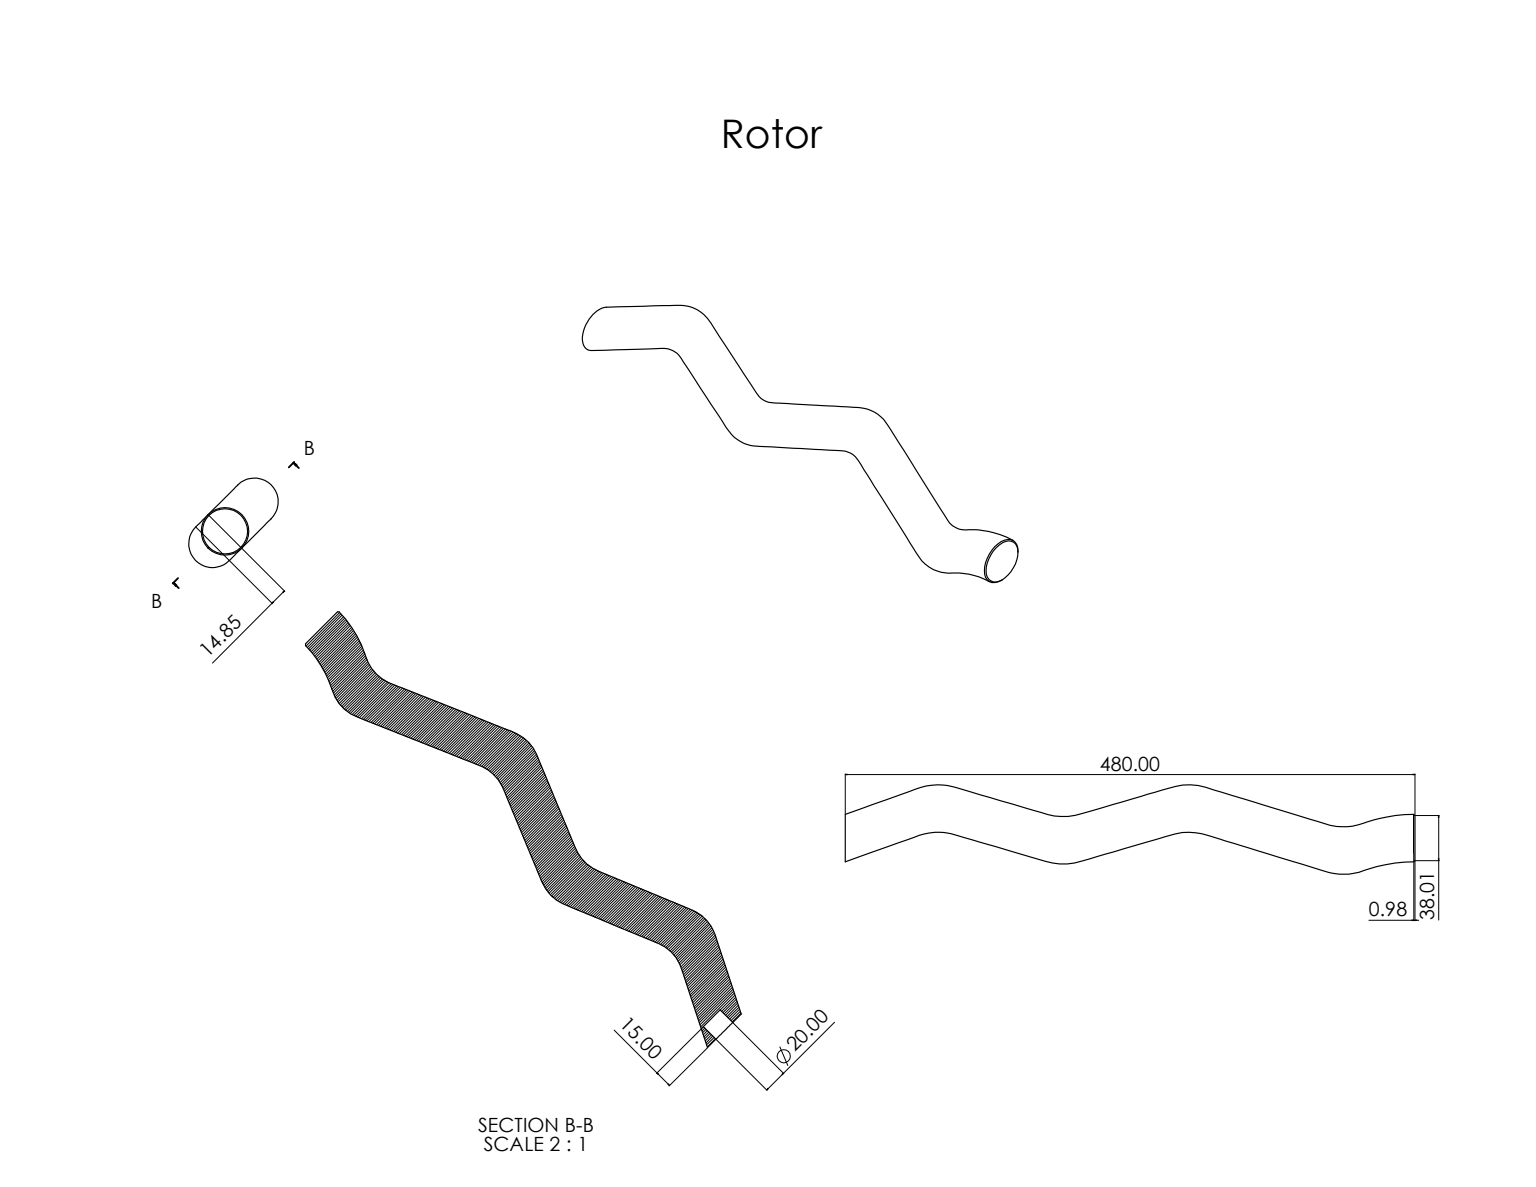
ISO-10303-21;
HEADER;
FILE_DESCRIPTION (('STEP AP214'),
    '1' );
FILE_NAME ('Rotor.step',
    '2026-10-27T19:20:31',
    ( '' ),
    ( '' ),
    'SwSTEP 2.0',
    'SolidWorks 2025',
    '' );
FILE_SCHEMA (( 'AUTOMOTIVE_DESIGN' ));
ENDSEC;

DATA;
#22=DIRECTION ( 'NONE',  ( 0.000000000000000000, 0.000000000000000000, 1.000000000000000000 ) ) ;
#25=CARTESIAN_POINT ( 'NONE',  ( 199.9999999999999432, 19.00168160052138333, -0.2996653188340382967 ) ) ;
#31=CARTESIAN_POINT ( 'NONE',  ( 199.0062801237116332, 7.031410157601610145, -18.72090521856086198 ) ) ;
#36=CARTESIAN_POINT ( 'NONE',  ( 200.0000000000002274, -16.15590588650048787, 10.03807108387658786 ) ) ;
#39=CARTESIAN_POINT ( 'NONE',  ( 199.0246859915949642, -4.071254240408448410, 19.58630271169732140 ) ) ;
#70=CARTESIAN_POINT ( 'NONE',  ( 200.0000000000001421, 16.62132632430557777, -9.210632111445709924 ) ) ;
#71=CARTESIAN_POINT ( 'NONE',  ( 199.9999999999999432, -18.84870794256249482, 2.485603278128234450 ) ) ;
#80=CARTESIAN_POINT ( 'NONE',  ( 199.0199757207951734, 7.646550829590152532, 18.48267855362066214 ) ) ;
#81=CARTESIAN_POINT ( 'NONE',  ( -100.7734535825088358, 12.25131212657497848, -12.25131212657469604 ) ) ;
#83=CARTESIAN_POINT ( 'NONE',  ( 19.06497207195980792, 66.60410523465830579, -10.03556273973354251 ) ) ;
#93=CARTESIAN_POINT ( 'NONE',  ( 199.9999999999998863, -17.04947422730185025, -8.406841951002201441 ) ) ;
#96=CARTESIAN_POINT ( 'NONE',  ( 199.0132273568269170, -10.00203194272371476, -17.32088655864767190 ) ) ;
#122=VERTEX_POINT ( 'NONE', #3583 ) ;
#126=SHAPE_REPRESENTATION ( 'Rotor', ( #21058 ), #20184 ) ;
#127=CARTESIAN_POINT ( 'NONE',  ( 199.9999999999999432, 17.49244587396685091, 7.427265670988617785 ) ) ;
#133=CARTESIAN_POINT ( 'NONE',  ( -259.2033419157646676, 21.55415060305860209, -21.55415060305812602 ) ) ;
#134=CARTESIAN_POINT ( 'NONE',  ( 199.0221265002223845, 3.088699012602908578, 19.76381171561452632 ) ) ;
#159=CARTESIAN_POINT ( 'NONE',  ( 199.9999999999999716, 8.674762155946922348, 16.91470172953081885 ) ) ;
#165=CARTESIAN_POINT ( 'NONE',  ( 199.0071786209885261, 3.739031945787267386, -19.64359944086908527 ) ) ;
#172=CARTESIAN_POINT ( 'NONE',  ( 199.0185982156405089, 10.13449990482401297, 17.24443922940779927 ) ) ;
#197=CARTESIAN_POINT ( 'NONE',  ( 200.0000000000001705, 18.83917254958691601, 2.502331228272203223 ) ) ;
#200=CARTESIAN_POINT ( 'NONE',  ( 199.9999999999999716, -19.00887936793599664, -0.3109487220520843476 ) ) ;
#209=CARTESIAN_POINT ( 'NONE',  ( 199.0242990326260042, -2.747623036511753991, 19.85784534697798875 ) ) ;
#210=CARTESIAN_POINT ( 'NONE',  ( 0.2972598230769959993, 38.42060263243713081, -38.42060263243619289 ) ) ;
#212=CARTESIAN_POINT ( 'NONE',  ( 146.6084372240433709, 3.800685668858042821, 52.76785682606522698 ) ) ;
#224=CARTESIAN_POINT ( 'NONE',  ( 199.0143331921596257, -11.79252763263196613, -16.15335214697885391 ) ) ;
#255=ORIENTED_EDGE ( 'NONE', *, *, #15646, .F. ) ;
#256=CARTESIAN_POINT ( 'NONE',  ( 199.9999999999998295, 18.60987205011830881, -3.837998380785754726 ) ) ;
#263=CARTESIAN_POINT ( 'NONE',  ( -208.1127848780265026, 10.60833733269551615, -10.60833733269529766 ) ) ;
#264=CARTESIAN_POINT ( 'NONE',  ( 199.0256575778758474, -7.963596585350240176, 18.35421432800287533 ) ) ;
#289=CARTESIAN_POINT ( 'NONE',  ( 199.9999999999999716, 17.03617407744741641, 8.421988063785285306 ) ) ;
#298=CARTESIAN_POINT ( 'NONE',  ( 199.0116000645839449, -7.055149577161559549, -18.71482085160166875 ) ) ;
#311=CARTESIAN_POINT ( 'NONE',  ( 199.0082178062215803, 19.99654772287713911, -0.6402344634765599896 ) ) ;
#337=CARTESIAN_POINT ( 'NONE',  ( 199.9999999999997442, 8.817246258963736594, -16.83121203733840332 ) ) ;
#338=CARTESIAN_POINT ( 'NONE',  ( 200.0000000000000284, -8.412522034014145333, -17.05141207210294851 ) ) ;
#349=CARTESIAN_POINT ( 'NONE',  ( 184.8905102610680444, 41.77492675555983936, 14.79361573936436081 ) ) ;
#351=CARTESIAN_POINT ( 'NONE',  ( 0.2972598230769886718, 38.42060263243643448, 18.14793986248763957 ) ) ;
#365=CARTESIAN_POINT ( 'NONE',  ( 199.0262399469797572, -16.26902294624164469, 11.64593733880351500 ) ) ;
#396=CARTESIAN_POINT ( 'NONE',  ( 199.9999999999997726, 10.29466221862743680, -15.97248499526360987 ) ) ;
#403=CARTESIAN_POINT ( 'NONE',  ( 136.1360204305621551, -53.05693388239309627, -3.511608612531332163 ) ) ;
#415=FACE_OUTER_BOUND ( 'NONE', #9966, .T. ) ;
#435=CARTESIAN_POINT ( 'NONE',  ( 199.0205186365099905, -18.88915341724846542, -6.581556047429298673 ) ) ;
#442=STYLED_ITEM('',(#26409),#26080);
#447=CARTESIAN_POINT ( 'NONE',  ( 199.0122446118616892, 18.20979473430505280, 8.267810710173087330 ) ) ;
#461=CARTESIAN_POINT ( 'NONE',  ( 199.0150639398586634, -12.88796719789325707, -15.29887847299889003 ) ) ;
#473=CARTESIAN_POINT ( 'NONE',  ( 199.9999999999999147, 7.974356211459238786, -17.24664066343551028 ) ) ;
#485=CARTESIAN_POINT ( 'NONE',  ( 14.38125909742181463, 10.73282306403652875, -67.30136555895941797 ) ) ;
#487=CARTESIAN_POINT ( 'NONE',  ( 91.82158438592158234, 16.11829626348378142, 40.45024623143977749 ) ) ;
#501=CARTESIAN_POINT ( 'NONE',  ( 200.0000000000000853, -10.31015863810315025, 15.97237410830284254 ) ) ;
#529=CARTESIAN_POINT ( 'NONE',  ( 199.9999999999997442, 17.78964944107278967, -6.681507572083275726 ) ) ;
#534=CARTESIAN_POINT ( 'NONE',  ( -162.0762913951021176, -27.08623940707584055, -29.48230308784799547 ) ) ;
#535=CARTESIAN_POINT ( 'NONE',  ( 199.0191753821509622, 9.128090787448098098, 17.79799345705162139 ) ) ;
#564=CARTESIAN_POINT ( 'NONE',  ( 199.9999999999999147, -2.490047575889294595, 18.88689753006142880 ) ) ;
#570=CARTESIAN_POINT ( 'NONE',  ( 199.0236444319429268, -19.98745889671670284, 0.8241971460415670192 ) ) ;
#581=CARTESIAN_POINT ( 'NONE',  ( 199.0103760074104002, 19.48024492545154018, 4.564568505664855280 ) ) ;
#595=CARTESIAN_POINT ( 'NONE',  ( 199.0058896134214024, 8.852588301136247395, -17.93157114668636964 ) ) ;
#605=CARTESIAN_POINT ( 'NONE',  ( 200.0000000000000000, 15.45062812681867825, -11.05917137904152625 ) ) ;
#616=CARTESIAN_POINT ( 'NONE',  ( 199.0138869583062728, 16.66122972709626637, 11.08110611611319740 ) ) ;
#617=CARTESIAN_POINT ( 'NONE',  ( -280.0000000000000568, -42.42640687119276066, -14.14213562373147148 ) ) ;
#633=CARTESIAN_POINT ( 'NONE',  ( 199.0262887415137527, -15.87643591937917442, 12.17243215972436055 ) ) ;
#660=CARTESIAN_POINT ( 'NONE',  ( 199.9999999999999432, 6.681520191215184035, -17.78964488229654251 ) ) ;
#664=CARTESIAN_POINT ( 'NONE',  ( 199.0161420530203600, 13.89456085230456850, 14.38651294782529888 ) ) ;
#695=CARTESIAN_POINT ( 'NONE',  ( 199.9999999999999147, 3.087032903897462432, 18.75855398088509318 ) ) ;
#701=CARTESIAN_POINT ( 'NONE',  ( 199.0171635947087907, -15.67013318013508716, -12.42972081464992407 ) ) ;
#705=AXIS2_PLACEMENT_3D ( 'NONE', #5212, #19434, #1220 ) ;
#715=CARTESIAN_POINT ( 'NONE',  ( 199.0068072339493597, 19.36029496603142874, -5.002335373038918398 ) ) ;
#731=CARTESIAN_POINT ( 'NONE',  ( 199.0058341074146142, 9.150281110520873895, -17.78147227136547670 ) ) ;
#733=ORIENTED_EDGE ( 'NONE', *, *, #5255, .F. ) ;
#743=CARTESIAN_POINT ( 'NONE',  ( 199.9999999999999432, 6.681520191215184035, -17.78964488229654251 ) ) ;
#744=CARTESIAN_POINT ( 'NONE',  ( 199.9999999999999147, -5.229706238425958276, -18.27161031230872368 ) ) ;
#752=CARTESIAN_POINT ( 'NONE',  ( 199.0072939989582324, 19.72179417679889823, -3.362695692811099590 ) ) ;
#753=CARTESIAN_POINT ( 'NONE',  ( -56.48582580120559271, -6.472252184284276844, 6.472252184284108978 ) ) ;
#767=CARTESIAN_POINT ( 'NONE',  ( 199.0263606093525652, -14.93202714917829965, 13.31409215216611663 ) ) ;
#796=CARTESIAN_POINT ( 'NONE',  ( 200.0000000000003126, 10.03286793820859835, -16.13825081434616493 ) ) ;
#799=CARTESIAN_POINT ( 'NONE',  ( 146.6084372240433709, -52.76785682606510619, -3.800685668859292043 ) ) ;
#800=CARTESIAN_POINT ( 'NONE',  ( 199.0185982156405089, 10.13449990482401297, 17.24443922940779927 ) ) ;
#815=CARTESIAN_POINT ( 'NONE',  ( -280.0000000000000000, -14.14213562373118549, 14.14213562373078936 ) ) ;
#833=CARTESIAN_POINT ( 'NONE',  ( 199.0220583073800640, -19.74674823417053915, -3.257374120286249397 ) ) ;
#844=CARTESIAN_POINT ( 'NONE',  ( 199.0053210531128229, 14.60061869579413063, -13.67646033072836786 ) ) ;
#860=CARTESIAN_POINT ( 'NONE',  ( 199.0089017020823121, -1.168865339877916965, -19.99575268797839911 ) ) ;
#872=CARTESIAN_POINT ( 'NONE',  ( 199.9999999999996021, 9.500464834803043601, -16.45734938164063621 ) ) ;
#873=CARTESIAN_POINT ( 'NONE',  ( 199.9999999999999432, 2.163685940895884841, -18.88015187541845918 ) ) ;
#883=CARTESIAN_POINT ( 'NONE',  ( 199.0119004238765967, 18.48644426806060181, 7.626980851762527713 ) ) ;
#885=CARTESIAN_POINT ( 'NONE',  ( -91.56559293963834989, -16.03295912088728414, 16.03295912088688269 ) ) ;
#898=CARTESIAN_POINT ( 'NONE',  ( 200.0000000000000000, -12.54535540268124372, 14.29661512548269187 ) ) ;
#925=CARTESIAN_POINT ( 'NONE',  ( 199.9999999999999716, -3.557237102606629620, -18.66704445460036865 ) ) ;
#929=CARTESIAN_POINT ( 'NONE',  ( 199.0091071337781159, 19.93120984291649478, 1.649067560610785854 ) ) ;
#943=CARTESIAN_POINT ( 'NONE',  ( 199.0250816517838359, -5.508431349499541163, 19.23181920140171997 ) ) ;
#946=CARTESIAN_POINT ( 'NONE',  ( 151.7948205124836534, 4.785054706297857230, 51.78348778862544322 ) ) ;
#963=CARTESIAN_POINT ( 'NONE',  ( 199.0254590212676078, -18.72437106667806717, 7.049340093992902290 ) ) ;
#990=CARTESIAN_POINT ( 'NONE',  ( 199.0112255263369718, -6.317613805557628304, -18.97682060292212114 ) ) ;
#1000=CARTESIAN_POINT ( 'NONE',  ( 199.9999999999999147, -10.82539530975288855, -15.62049148088690131 ) ) ;
#1010=CARTESIAN_POINT ( 'NONE',  ( -213.1075012329537230, 9.698598906450543566, -9.698598906450348167 ) ) ;
#1027=CARTESIAN_POINT ( 'NONE',  ( 199.9999999999999716, 2.158921371974932057, 18.88613560767030464 ) ) ;
#1051=CARTESIAN_POINT ( 'NONE',  ( 200.0000000000000568, 2.475862818518347552, -18.83975305017670365 ) ) ;
#1055=CARTESIAN_POINT ( 'NONE',  ( 199.0190933210857906, 9.274233341078666371, 17.72222919763310856 ) ) ;
#1069=CARTESIAN_POINT ( 'NONE',  ( 0.2972598230769938343, 10.13633138497486286, -10.13633138497461594 ) ) ;
#1084=CARTESIAN_POINT ( 'NONE',  ( 200.0000000000000568, 3.396018298074437780, 18.70303282425911462 ) ) ;
#1122=CARTESIAN_POINT ( 'NONE',  ( -265.0000000000000000, -4.867971026610730343E-14, -6.532754371361504014E-30 ) ) ;
#1132=CARTESIAN_POINT ( 'NONE',  ( 199.9999999999994031, -18.37269623729978107, -4.912321869774860517 ) ) ;
#1157=CARTESIAN_POINT ( 'NONE',  ( 200.0000000000003695, 4.006257452897062699, 18.58368358710308144 ) ) ;
#1182=CARTESIAN_POINT ( 'NONE',  ( 199.9999999999999147, -13.00175152101318510, -13.87559618198639022 ) ) ;
#1185=CARTESIAN_POINT ( 'NONE',  ( 199.0075387591496110, 2.605640672139595715, -19.82598477556707195 ) ) ;
#1206=( LENGTH_UNIT ( ) NAMED_UNIT ( * ) SI_UNIT ( .MILLI., .METRE. ) );
#1215=CARTESIAN_POINT ( 'NONE',  ( 200.0000000000000853, -10.31015863810315025, 15.97237410830284254 ) ) ;
#1220=DIRECTION ( 'NONE',  ( 0.000000000000000000, -1.000000000000000000, 0.000000000000000000 ) ) ;
#1243=CARTESIAN_POINT ( 'NONE',  ( 199.0233014162839140, -20.00325696956714339, -0.1274617848538161236 ) ) ;
#1251=CARTESIAN_POINT ( 'NONE',  ( 136.1360204305621266, 3.511608612530757068, -3.511608612530642937 ) ) ;
#1253=CARTESIAN_POINT ( 'NONE',  ( 199.9999999999998010, -18.94725682776174835, -1.557189005449375330 ) ) ;
#1277=CARTESIAN_POINT ( 'NONE',  ( 199.9999999999998295, 8.812783067309094776, 16.84096882534935702 ) ) ;
#1304=CARTESIAN_POINT ( 'NONE',  ( 199.9999999999996305, -13.87326568555608830, -12.99368172854615366 ) ) ;
#1307=CARTESIAN_POINT ( 'NONE',  ( 199.0053384867209445, 15.04244419640346031, -13.18878631234924192 ) ) ;
#1328=CARTESIAN_POINT ( 'NONE',  ( -86.96347745069644475, -15.38646221621807442, 15.38646221621768184 ) ) ;
#1333=ORIENTED_EDGE ( 'NONE', *, *, #17104, .F. ) ;
#1339=CARTESIAN_POINT ( 'NONE',  ( 200.0000000000003411, -11.08347333911627963, 15.44584840147742355 ) ) ;
#1349=B_SPLINE_CURVE_WITH_KNOTS ( 'NONE', 3,
 ( #13548, #17297, #15539, #5314, #1457, #9433, #11058, #13425, #21548, #7058, #19543, #17540, #1328, #7425, #25678, #23667, #21301, #5447, #9184, #21801, #9691, #7684, #17797, #23922, #3574, #13679, #15798, #25943, #11677, #19802 ),
 .UNSPECIFIED., .F., .F.,
 ( 4, 2, 2, 2, 2, 2, 2, 2, 2, 2, 2, 2, 2, 2, 4 ),
 ( 0.000000000000000000, 0.1357259735107005372, 0.1651108541090157700, 0.1944957347073310028, 0.3598804999793158710, 0.3867117631979620773, 0.4135430264166082281, 0.5789277916885930964, 0.6062785021374117456, 0.6336292125862302838, 0.8508620842112317728, 0.8814014469398914198, 0.9119408096685510667, 0.9559704048342755334, 0.9981086137545830406 ),
 .UNSPECIFIED. ) ;
#1384=CARTESIAN_POINT ( 'NONE',  ( 199.9999999999999716, -15.72304121538119936, -10.67928908684366540 ) ) ;
#1410=CARTESIAN_POINT ( 'NONE',  ( 200.0000000000000568, -6.707298731100607370, 17.79007541258576452 ) ) ;
#1434=CARTESIAN_POINT ( 'NONE',  ( 200.0000000000000000, -10.04040541317802315, -16.13598245992451297 ) ) ;
#1438=CARTESIAN_POINT ( 'NONE',  ( 199.0055466334479206, 16.72508833076945223, -10.95857635003404873 ) ) ;
#1457=CARTESIAN_POINT ( 'NONE',  ( -208.1127848780265026, 10.60833733269551615, -10.60833733269529766 ) ) ;
#1467=CARTESIAN_POINT ( 'NONE',  ( 199.9999999999998863, -2.178116022715518074, 18.88665387132288487 ) ) ;
#1468=CARTESIAN_POINT ( 'NONE',  ( -280.0000000000000000, 14.14213562373108424, -14.14213562373078759 ) ) ;
#1500=CARTESIAN_POINT ( 'NONE',  ( 199.0198738297864338, -18.40122271749203620, -7.840790799891646401 ) ) ;
#1502=ORIENTED_EDGE ( 'NONE', *, *, #5255, .T. ) ;
#1508=CARTESIAN_POINT ( 'NONE',  ( -208.1127848780265026, 38.89260858015777700, -38.89260858015687461 ) ) ;
#1511=CARTESIAN_POINT ( 'NONE',  ( 199.9999999999998579, -17.31468161508541570, -7.846489601088847188 ) ) ;
#1526=CARTESIAN_POINT ( 'NONE',  ( 184.8905102610680444, -14.79361573936399665, 14.79361573936367158 ) ) ;
#1541=CARTESIAN_POINT ( 'NONE',  ( 199.9999999999998579, 3.088973468740698447, 18.75625871509165776 ) ) ;
#1554=CARTESIAN_POINT ( 'NONE',  ( 57.59792236341147031, 26.56190807104652052, 30.00663442387728708 ) ) ;
#1566=CARTESIAN_POINT ( 'NONE',  ( 200.0000000000000568, -15.63904601878861733, 10.81246610429574595 ) ) ;
#1569=CARTESIAN_POINT ( 'NONE',  ( 199.0059805750804571, 8.391908656364034158, -18.14947886101857932 ) ) ;
#1600=CARTESIAN_POINT ( 'NONE',  ( 199.9999999999996874, -6.995992324030534171, 17.67857064404661926 ) ) ;
#1606=CARTESIAN_POINT ( 'NONE',  ( 0.2972598230769959993, 38.42060263243713081, -38.42060263243619289 ) ) ;
#1642=CARTESIAN_POINT ( 'NONE',  ( 91.82158438592158234, 16.11829626346161604, -16.11829626346121103 ) ) ;
#1660=AXIS2_PLACEMENT_3D ( 'NONE', #24424, #14168, #4078 ) ;
#1671=FACE_OUTER_BOUND ( 'NONE', #18068, .T. ) ;
#1672=CARTESIAN_POINT ( 'NONE',  ( 199.9999999999998863, 18.50936851023984886, -4.296315843485498220 ) ) ;
#1675=CARTESIAN_POINT ( 'NONE',  ( 199.9999999999999432, -18.10102589806735907, -5.808760618774897466 ) ) ;
#1687=CARTESIAN_POINT ( 'NONE',  ( 184.8905102610680444, -14.79361573936399665, 14.79361573936367158 ) ) ;
#1690=CARTESIAN_POINT ( 'NONE',  ( 57.59792236341147031, -1.722363176415055985, 1.722363176415024677 ) ) ;
#1703=CARTESIAN_POINT ( 'NONE',  ( 199.0069448139248891, 19.47830345430216070, -4.521371627647083891 ) ) ;
#1729=CARTESIAN_POINT ( 'NONE',  ( 200.0000000000000284, 10.29196162618721644, 15.98165385515595815 ) ) ;
#1735=CARTESIAN_POINT ( 'NONE',  ( -56.48582580120559982, -6.472252184283581400, -50.09629031063973059 ) ) ;
#1736=CYLINDRICAL_SURFACE ( 'NONE', #23013, 10.00000000000000000 ) ;
#1762=CARTESIAN_POINT ( 'NONE',  ( 200.0000000000000000, 18.75319608166667251, -3.074485549213874069 ) ) ;
#1770=CARTESIAN_POINT ( 'NONE',  ( 199.0064300168743898, 6.416848550863170964, -18.94043562797172697 ) ) ;
#1781=CARTESIAN_POINT ( 'NONE',  ( 199.0160554649137907, 14.01242985958090692, 14.27167877623515757 ) ) ;
#1806=CARTESIAN_POINT ( 'NONE',  ( 199.0053211798077086, 14.13837298227953987, -14.13837298578013701 ) ) ;
#1807=CARTESIAN_POINT ( 'NONE',  ( 199.9999999999999432, 16.89472078740815775, 8.702431973737679627 ) ) ;
#1808=CARTESIAN_POINT ( 'NONE',  ( 199.9999999999999147, -18.88644897276319412, 2.180134100127611330 ) ) ;
#1818=CARTESIAN_POINT ( 'NONE',  ( 199.0148629966199962, 15.54375530361796010, 12.59047442983698417 ) ) ;
#1820=CARTESIAN_POINT ( 'NONE',  ( -100.7734535825088500, -16.03295912088659492, -40.53558337403696044 ) ) ;
#1823=CARTESIAN_POINT ( 'NONE',  ( -192.9588430854689989, 10.23066800230756712, -10.23066800230735396 ) ) ;
#1834=CARTESIAN_POINT ( 'NONE',  ( 199.9999999999999147, -18.99336422956244874, -0.7807574862979690389 ) ) ;
#1837=CARTESIAN_POINT ( 'NONE',  ( 199.0183492910935286, -16.99256592298258184, -10.55490704374186883 ) ) ;
#1867=CARTESIAN_POINT ( 'NONE',  ( 199.9999999999998863, 8.252615397115851792, 17.12261885615216173 ) ) ;
#1873=CARTESIAN_POINT ( 'NONE',  ( -30.26275506840323715, 29.48230279907829754, -29.48230279907758344 ) ) ;
#1874=CARTESIAN_POINT ( 'NONE',  ( 199.0245441510845410, -3.586860678693493565, 19.68275873856094549 ) ) ;
#1898=CARTESIAN_POINT ( 'NONE',  ( 199.9999999999999432, 17.99863635774381621, -6.096428138147773623 ) ) ;
#1905=CARTESIAN_POINT ( 'NONE',  ( 199.0078712948245823, 1.622169390422157242, -19.93073376281416031 ) ) ;
#1912=CARTESIAN_POINT ( 'NONE',  ( 199.0218477376944577, 3.734929907270702287, 19.65178994764128717 ) ) ;
#1939=CARTESIAN_POINT ( 'NONE',  ( 200.0000000000005116, 16.46820326627658204, -9.481692438271846157 ) ) ;
#1940=CARTESIAN_POINT ( 'NONE',  ( 199.9999999999999432, -18.70500695855449891, 3.403006402435800215 ) ) ;
#1943=CARTESIAN_POINT ( 'NONE',  ( -100.7734535825088500, -16.03295912088659492, -40.53558337403696044 ) ) ;
#1950=CARTESIAN_POINT ( 'NONE',  ( 199.0255783348552825, -7.592917736791534367, 18.50773992579789251 ) ) ;
#1951=CARTESIAN_POINT ( 'NONE',  ( 200.0000000000000000, 42.42640687119267540, 14.14213562373153543 ) ) ;
#1966=CARTESIAN_POINT ( 'NONE',  ( 200.0000000000001137, -18.36608873747554327, 4.914565663504686377 ) ) ;
#1970=CARTESIAN_POINT ( 'NONE',  ( 199.0201284062958962, -18.60237515726647572, -7.352601386804158423 ) ) ;
#1987=SHAPE_DEFINITION_REPRESENTATION ( #9744, #126 ) ;
#1996=CARTESIAN_POINT ( 'NONE',  ( 199.9999999999995737, 11.06459441337805494, 15.46579378046570952 ) ) ;
#2004=CARTESIAN_POINT ( 'NONE',  ( 184.8905102610680444, -14.79361573936330565, -41.77492675556016621 ) ) ;
#2005=CARTESIAN_POINT ( 'NONE',  ( 199.0247325273615502, -4.232801689760709252, 19.55205092890061280 ) ) ;
#2034=CARTESIAN_POINT ( 'NONE',  ( 199.9999999999999432, 12.28098720308154945, 14.50824971548827946 ) ) ;
#2040=CARTESIAN_POINT ( 'NONE',  ( 199.0075387591496110, 2.605640672139595715, -19.82598477556707195 ) ) ;
#2045=CARTESIAN_POINT ( 'NONE',  ( 200.0000000000001990, -15.46007656673369368, 11.06691610098113543 ) ) ;
#2048=CARTESIAN_POINT ( 'NONE',  ( 199.0248683625651154, -4.715036670046848677, 19.44145415004932076 ) ) ;
#2072=DIRECTION ( 'NONE',  ( -1.000000000000000000, -1.836970198721030181E-16, -2.465190328815661892E-32 ) ) ;
#2073=CARTESIAN_POINT ( 'NONE',  ( 199.9999999999999716, 17.67160698027466736, 6.995183481556395577 ) ) ;
#2074=CARTESIAN_POINT ( 'NONE',  ( 199.9999999999998863, -18.51554692031677973, -4.309913066855557418 ) ) ;
#2083=CARTESIAN_POINT ( 'NONE',  ( 199.0253317321493398, -6.507757088401906032, 18.91903323328891062 ) ) ;
#2085=CARTESIAN_POINT ( 'NONE',  ( -238.4067589809705794, 0.6820004458491113475, -57.25054294077229144 ) ) ;
#2087=CARTESIAN_POINT ( 'NONE',  ( -162.0762913951021176, 57.76657433523994456, -1.198031840315424867 ) ) ;
#2096=CARTESIAN_POINT ( 'NONE',  ( 199.9999999999998579, -15.18157530797039101, 11.44282300742696457 ) ) ;
#2100=CARTESIAN_POINT ( 'NONE',  ( 199.0125641721520822, -8.847877585088737007, -17.93749959268865979 ) ) ;
#2119=ORIENTED_EDGE ( 'NONE', *, *, #8406, .T. ) ;
#2128=CARTESIAN_POINT ( 'NONE',  ( 199.9999999999999432, 17.03543292729471403, 8.423468753378063667 ) ) ;
#2134=CARTESIAN_POINT ( 'NONE',  ( -135.8532207217289738, 21.81201906317798134, -21.81201906317747685 ) ) ;
#2135=CARTESIAN_POINT ( 'NONE',  ( 199.0258842571097375, -9.142960865851959440, 17.79628948870135829 ) ) ;
#2162=CARTESIAN_POINT ( 'NONE',  ( 200.0000000000000000, 9.495512316542487952, 16.46764514154290637 ) ) ;
#2169=CARTESIAN_POINT ( 'NONE',  ( 199.0057329523134513, 9.713090712928652337, -17.48024697358846069 ) ) ;
#2176=CARTESIAN_POINT ( 'NONE',  ( 199.9999999999998863, -17.44218472118251384, 7.566354988273278792 ) ) ;
#2179=CARTESIAN_POINT ( 'NONE',  ( 199.0212010157159455, 5.167062836304152640, 19.32642926518865423 ) ) ;
#2206=CARTESIAN_POINT ( 'NONE',  ( 199.9999999999997442, 18.75350838795884201, -3.072479883316599381 ) ) ;
#2207=CARTESIAN_POINT ( 'NONE',  ( 199.9999999999999147, -11.57906590988528528, -15.07304842808868273 ) ) ;
#2210=CARTESIAN_POINT ( 'NONE',  ( -280.0000000000000000, -5.143516556418885689E-14, 0.000000000000000000 ) ) ;
#2216=CARTESIAN_POINT ( 'NONE',  ( 199.0260505877926960, -10.07036125175988772, 17.33556466753674385 ) ) ;
#2217=CARTESIAN_POINT ( 'NONE',  ( 19.06497207195980792, 66.60410523465830579, -10.03556273973354251 ) ) ;
#2219=CARTESIAN_POINT ( 'NONE',  ( -198.0356074513804572, 39.15871834505887250, 17.40982414986519089 ) ) ;
#2231=CARTESIAN_POINT ( 'NONE',  ( 199.0178460907175690, -16.45326163792621443, -11.37340206338170923 ) ) ;
#2258=CARTESIAN_POINT ( 'NONE',  ( 200.0000000000001137, 17.30391983412833667, 7.856783789979721710 ) ) ;
#2264=CARTESIAN_POINT ( 'NONE',  ( 4.995406935893294431, -17.50105314357144337, -39.06748935135212264 ) ) ;
#2265=DIRECTION ( 'NONE',  ( -1.000000000000000000, -1.836970198721030181E-16, -2.465190328815661892E-32 ) ) ;
#2280=EDGE_LOOP ( 'NONE', ( #12322, #25337 ) ) ;
#2288=CARTESIAN_POINT ( 'NONE',  ( 199.9999999999999147, 18.96428544249645043, -1.225771028434774923 ) ) ;
#2293=CARTESIAN_POINT ( 'NONE',  ( 199.0060750228415429, 7.941611777091910795, -18.35102805502410561 ) ) ;
#2297=CARTESIAN_POINT ( 'NONE',  ( -280.0000000000000000, -5.143516556418885689E-14, 0.000000000000000000 ) ) ;
#2303=CARTESIAN_POINT ( 'NONE',  ( 199.0201394418415077, 7.332745681712491859, 18.61237044096938575 ) ) ;
#2331=CARTESIAN_POINT ( 'NONE',  ( 200.0000000000000000, 2.939587388390868306, -18.77290383772223592 ) ) ;
#2332=CARTESIAN_POINT ( 'NONE',  ( 199.9999999999999716, -2.174716591481574035, -18.87967999152925103 ) ) ;
#2343=CARTESIAN_POINT ( 'NONE',  ( 199.0193791362118532, 8.756460839110824068, 17.98522136602180055 ) ) ;
#2344=CARTESIAN_POINT ( 'NONE',  ( 4.995406935893286438, 67.35176059880245703, -10.78321810387767066 ) ) ;
#2346=CARTESIAN_POINT ( 'NONE',  ( -100.7734535825088500, 12.25131212657428748, 44.31723036834913643 ) ) ;
#2360=CARTESIAN_POINT ( 'NONE',  ( 199.0130599948309680, -9.716555752287060699, -17.48250520384952367 ) ) ;
#2388=CARTESIAN_POINT ( 'NONE',  ( 199.9999999999996021, 4.009690090792337180, -18.57554820616829261 ) ) ;
#2394=CARTESIAN_POINT ( 'NONE',  ( 184.8905102610680444, -43.07788698682556827, -13.49065550809859104 ) ) ;
#2395=CARTESIAN_POINT ( 'NONE',  ( 199.0262120803540995, -11.39568569719682145, 16.44280778893389439 ) ) ;
#2408=CARTESIAN_POINT ( 'NONE',  ( 199.0261461916015264, -10.84957391917088110, 16.80813345823991867 ) ) ;
#2422=CARTESIAN_POINT ( 'NONE',  ( 199.9999999999999716, -6.125576256895536531, 18.00661530747469996 ) ) ;
#2428=CARTESIAN_POINT ( 'NONE',  ( 199.0198127172867828, -18.35326955327933618, -7.958687714023728432 ) ) ;
#2436=CARTESIAN_POINT ( 'NONE',  ( -265.0000000000000000, -4.867971026610730343E-14, -6.532754371361504014E-30 ) ) ;
#2437=CARTESIAN_POINT ( 'NONE',  ( 199.0066757862822726, 19.23093628729661475, -5.478378800400602877 ) ) ;
#2450=APPLICATION_CONTEXT ( 'automotive_design' ) ;
#2452=CARTESIAN_POINT ( 'NONE',  ( 199.0118788846117468, -7.586312082139164303, -18.50318004405354699 ) ) ;
#2464=CARTESIAN_POINT ( 'NONE',  ( 200.0000000000001137, 15.89309473284322749, -10.41337480477382371 ) ) ;
#2474=CARTESIAN_POINT ( 'NONE',  ( 199.0112297511867325, 18.97400286213774834, 6.326091761587574247 ) ) ;
#2475=CARTESIAN_POINT ( 'NONE',  ( 163.1118516004056573, -47.56205970284945295, -9.006482792074823607 ) ) ;
#2477=CARTESIAN_POINT ( 'NONE',  ( 0.2972598230769907257, 66.70487387989869887, -10.13633138497392494 ) ) ;
#2493=CARTESIAN_POINT ( 'NONE',  ( 199.9999999999997158, -10.44119114510941770, 15.88703355754643098 ) ) ;
#2523=CARTESIAN_POINT ( 'NONE',  ( 199.9999999999998863, 12.52392839731578889, -14.30162278802013098 ) ) ;
#2526=CARTESIAN_POINT ( 'NONE',  ( 130.8568914410475372, -24.07718906447255947, 24.07718906447199458 ) ) ;
#2527=CARTESIAN_POINT ( 'NONE',  ( 199.0117592729713465, 18.59672480091233737, 7.361113620700817428 ) ) ;
#2554=CARTESIAN_POINT ( 'NONE',  ( 199.9999999999999716, -10.82917866272351581, 15.62749623992054637 ) ) ;
#2561=CARTESIAN_POINT ( 'NONE',  ( 199.0234688043258018, -20.00162938710794691, 0.3307560783973806373 ) ) ;
#2575=CARTESIAN_POINT ( 'NONE',  ( 199.0055623607443636, 10.83365079593514757, -16.80863377785637169 ) ) ;
#2590=CARTESIAN_POINT ( 'NONE',  ( 199.0118983629657237, -7.623092896147099395, -18.48804935406682404 ) ) ;
#2602=CARTESIAN_POINT ( 'NONE',  ( 199.9999999999997726, 7.546454185142647653, -17.43816512261951956 ) ) ;
#2603=CARTESIAN_POINT ( 'NONE',  ( 199.9999999999999147, 4.913383178421502073, -18.36491317384603761 ) ) ;
#2613=CARTESIAN_POINT ( 'NONE',  ( 199.0063941363436584, 18.94647080546362261, -6.505566240119136090 ) ) ;
#2614=CARTESIAN_POINT ( 'NONE',  ( 130.8568914410475088, -52.36146031193413108, -4.207082182990267150 ) ) ;
#2633=CARTESIAN_POINT ( 'NONE',  ( 199.0262772983307400, -15.97594543884460450, 12.04151787815577102 ) ) ;
#2663=CARTESIAN_POINT ( 'NONE',  ( 199.9999999999999147, 7.974356211459238786, -17.24664066343551028 ) ) ;
#2668=CARTESIAN_POINT ( 'NONE',  ( 199.0194208361885444, 8.684746017668368623, 18.01861981654000999 ) ) ;
#2695=( NAMED_UNIT ( * ) SI_UNIT ( $, .STERADIAN. ) SOLID_ANGLE_UNIT ( ) );
#2698=CARTESIAN_POINT ( 'NONE',  ( 199.9999999999999432, 5.207736135262080346, 18.28309964035191726 ) ) ;
#2704=CARTESIAN_POINT ( 'NONE',  ( 199.0181825105790665, -16.81808889125263207, -10.83063377519274795 ) ) ;
#2715=CARTESIAN_POINT ( 'NONE',  ( 199.0093797572272081, 19.86600527971208763, 2.306481033292959726 ) ) ;
#2729=CARTESIAN_POINT ( 'NONE',  ( 199.0053214113103763, 13.24708851623085870, -15.02902163144573500 ) ) ;
#2740=CARTESIAN_POINT ( 'NONE',  ( 199.9999999999997726, -2.174764995058875439, -18.87968408895515182 ) ) ;
#2741=CARTESIAN_POINT ( 'NONE',  ( 200.0000000000000000, -0.6316560126811792131, -18.99370827960111541 ) ) ;
#2750=CARTESIAN_POINT ( 'NONE',  ( 199.0114847477458397, 18.79655487626452981, 6.828771775710518632 ) ) ;
#2752=CARTESIAN_POINT ( 'NONE',  ( -238.4067589809705794, -27.60227080167029001, -28.96627169325357798 ) ) ;
#2766=CARTESIAN_POINT ( 'NONE',  ( 199.0230409161751197, -19.98726064469808961, -0.8218112272605428981 ) ) ;
#2793=CARTESIAN_POINT ( 'NONE',  ( 199.9999999999999716, 18.70067531203203970, -3.379044910449504169 ) ) ;
#2796=CARTESIAN_POINT ( 'NONE',  ( 0.2972598230769938343, 10.13633138497486286, -10.13633138497461594 ) ) ;
#2797=CARTESIAN_POINT ( 'NONE',  ( 199.0206025836015442, 6.413712542583970944, 18.94893284924772203 ) ) ;
#2834=CARTESIAN_POINT ( 'NONE',  ( 199.0145894657785846, -12.18649378798404470, -15.86093292504746621 ) ) ;
#2848=CARTESIAN_POINT ( 'NONE',  ( 199.0060751070798233, 18.35498561216385482, -7.937441424495496278 ) ) ;
#2874=CARTESIAN_POINT ( 'NONE',  ( 199.9999999999997726, 10.29466221862743680, -15.97248499526360987 ) ) ;
#2875=CARTESIAN_POINT ( 'NONE',  ( 199.9999999999999147, -6.120187099840395106, -17.99310556315726117 ) ) ;
#2883=CARTESIAN_POINT ( 'NONE',  ( 199.0060844782017000, 18.36908416490651064, -7.898827608825804703 ) ) ;
#2884=CARTESIAN_POINT ( 'NONE',  ( 170.2234770963711128, -17.36149277826940462, -39.20704971665412586 ) ) ;
#2898=CARTESIAN_POINT ( 'NONE',  ( 199.0254590212676078, -18.72437106667806717, 7.049340093992902290 ) ) ;
#2922=CARTESIAN_POINT ( 'NONE',  ( 199.9999999999999147, -6.121038220875967717, -17.99280653461927315 ) ) ;
#2926=CARTESIAN_POINT ( 'NONE',  ( 199.0173417939125784, 12.16728005963107329, 15.88742495833056800 ) ) ;
#2940=CARTESIAN_POINT ( 'NONE',  ( -100.7734535825088358, -16.03295912088728770, 16.03295912088687913 ) ) ;
#2952=CARTESIAN_POINT ( 'NONE',  ( 199.9999999999999716, -11.08296553609489798, 15.44857252758585631 ) ) ;
#2956=CARTESIAN_POINT ( 'NONE',  ( 199.0186803405091780, -17.32754287553631301, -9.995805879000721816 ) ) ;
#2986=CARTESIAN_POINT ( 'NONE',  ( 199.0053211804427633, 14.13331159297750617, -14.14343255912447361 ) ) ;
#2998=CARTESIAN_POINT ( 'NONE',  ( 200.0000000000000284, -14.89093438834758842, -11.81132417993805639 ) ) ;
#3007=CARTESIAN_POINT ( 'NONE',  ( 199.0094106630088220, 19.89429631425563372, 2.408647560944259691 ) ) ;
#3009=CARTESIAN_POINT ( 'NONE',  ( 170.2234770963711128, -45.64576402573167258, -10.92277846919254891 ) ) ;
#3023=CARTESIAN_POINT ( 'NONE',  ( 199.0053211798077086, 14.13837298227953987, -14.13837298578013701 ) ) ;
#3024=CARTESIAN_POINT ( 'NONE',  ( 200.0000000000001421, -10.70065846580424207, 15.71346033962178446 ) ) ;
#3047=CARTESIAN_POINT ( 'NONE',  ( 199.9999999999999147, 0.2978356717867484682, -19.00168788844713319 ) ) ;
#3050=CARTESIAN_POINT ( 'NONE',  ( 199.0082178062215803, 19.99654772287713911, -0.6402344634765599896 ) ) ;
#3067=CARTESIAN_POINT ( 'NONE',  ( 199.0258313909553749, -8.851116586292111066, 17.94317422212728630 ) ) ;
#3069=CARTESIAN_POINT ( 'NONE',  ( -213.1075012329537230, 37.98287015391211696, 18.58567234101190735 ) ) ;
#3086=CARTESIAN_POINT ( 'NONE',  ( 199.0263606093525652, -14.93202714917829965, 13.31409215216611663 ) ) ;
#3105=ORIENTED_EDGE ( 'NONE', *, *, #16287, .F. ) ;
#3111=CARTESIAN_POINT ( 'NONE',  ( 199.0230723762332161, -19.99042835476056368, -0.7383407320838223376 ) ) ;
#3122=CARTESIAN_POINT ( 'NONE',  ( 199.9999999999999716, -17.78976893299991247, -6.695511796223322598 ) ) ;
#3132=B_SPLINE_CURVE_WITH_KNOTS ( 'NONE', 3,
 ( #11253, #9647, #7634, #20030, #7906, #20159, #9911, #18285, #15883, #10316, #18017, #16025, #4211, #10181, #18422, #10048, #16297, #7768, #24295, #5789, #22434, #1940, #18154, #71, #1808, #26166, #12301, #200, #11907, #8307, #22298, #20428, #6185, #22167, #14165, #2074, #24009, #21886, #1675, #26301, #4074, #24150, #26031, #6313, #5927, #3942, #14034, #13896, #8044, #12039, #22030, #16432, #19890, #16160, #3663, #6063, #3803, #12176, #20297, #9780, #2207, #8180, #24421, #24558, #14300, #11771, #17882, #8848, #338, #16828, #12844, #4868, #2875, #10983, #744, #12565, #14962, #16691, #21095, #4734, #20960, #2332, #10575, #8442, #2741, #19093, #12972, #16958, #873, #14433, #8713, #23097, #22562, #6577, #2603, #24824, #18690, #12433, #18559, #25096, #8982, #6843, #17089, #10845, #25221, #4341, #16561, #24690, #20561, #10445, #20699, #12701, #6446, #14696, #14562 ),
 .UNSPECIFIED., .F., .F.,
 ( 4, 2, 1, 2, 2, 2, 2, 2, 1, 2, 2, 2, 2, 2, 2, 1, 2, 2, 2, 2, 2, 1, 2, 2, 2, 2, 2, 2, 2, 2, 2, 2, 2, 2, 1, 2, 2, 2, 2, 2, 2, 2, 2, 2, 2, 2, 2, 1, 2, 2, 2, 2, 2, 1, 2, 2, 2, 2, 2, 2, 4 ),
 ( 0.000000000000000000, 0.01562500000000010061, 0.02343750000000014572, 0.02734375000000015613, 0.03125000000000015959, 0.04687500000000018041, 0.05468750000000021511, 0.06250000000000024980, 0.07031250000000029143, 0.07421875000000027756, 0.07812500000000027756, 0.09375000000000033307, 0.1015625000000003608, 0.1093750000000003886, 0.1250000000000004441, 0.1328125000000004718, 0.1367187500000004718, 0.1406250000000004718, 0.1562500000000004996, 0.1640625000000005274, 0.1718750000000005551, 0.1796875000000005829, 0.1835937500000006106, 0.1875000000000006106, 0.2031250000000007494, 0.2109375000000008049, 0.2187500000000008604, 0.2265625000000009159, 0.2343750000000009437, 0.2421875000000009992, 0.2500000000000010547, 0.2656250000000012768, 0.2734375000000013878, 0.2812500000000014988, 0.2890625000000015543, 0.2929687500000015543, 0.2968750000000015543, 0.3125000000000014988, 0.3203125000000014433, 0.3281250000000013878, 0.3359375000000013323, 0.3437500000000012768, 0.3515625000000012212, 0.3593750000000011657, 0.3671875000000011102, 0.3750000000000009992, 0.3906250000000009437, 0.3984375000000008882, 0.4023437500000008882, 0.4062500000000008327, 0.4218750000000006661, 0.4296875000000005551, 0.4375000000000004441, 0.4453125000000003886, 0.4492187500000003331, 0.4531250000000003331, 0.4609375000000002220, 0.4687500000000001665, 0.4765625000000001110, 0.4843750000000000555, 0.5000000000000000000 ),
 .UNSPECIFIED. ) ;
#3148=CARTESIAN_POINT ( 'NONE',  ( 199.9999999999999716, 1.225499021177249404, 18.97167928969624384 ) ) ;
#3174=CARTESIAN_POINT ( 'NONE',  ( 199.9999999999999147, -4.475453068641236598, -18.46865746885900705 ) ) ;
#3177=CARTESIAN_POINT ( 'NONE',  ( 199.0073806320087613, 3.093635517344801578, -19.75563546371214230 ) ) ;
#3202=CARTESIAN_POINT ( 'NONE',  ( 199.0263771353516233, -14.14574067859894413, 14.14574067859863682 ) ) ;
#3235=CARTESIAN_POINT ( 'NONE',  ( 199.0255658961882830, -18.53135165341859292, 7.535237739358464637 ) ) ;
#3246=CARTESIAN_POINT ( 'NONE',  ( 200.0000000000001137, -7.564955314186367907, -17.43543124971759539 ) ) ;
#3274=CARTESIAN_POINT ( 'NONE',  ( 199.9999999999999716, 8.673909288817675645, 16.91296503504769078 ) ) ;
#3301=CARTESIAN_POINT ( 'NONE',  ( 199.9999999999998579, -2.482523633563583410, -18.84177167654976515 ) ) ;
#3304=CARTESIAN_POINT ( 'NONE',  ( 199.0057363775755448, 17.49143510765091492, -9.692886659233986180 ) ) ;
#3331=CARTESIAN_POINT ( 'NONE',  ( 199.0262110011730954, -16.45735938206000171, 11.37817034370231006 ) ) ;
#3355=CARTESIAN_POINT ( 'NONE',  ( 200.0000000000000000, -13.44239485489230290, 13.44239485489200803 ) ) ;
#3358=CARTESIAN_POINT ( 'NONE',  ( 199.0193679503813939, -17.97530889761664596, -8.776769756081623797 ) ) ;
#3369=CARTESIAN_POINT ( 'NONE',  ( 199.9999999999998863, -11.82502131081330887, -14.88093782183822888 ) ) ;
#3393=DIRECTION ( 'NONE',  ( -1.000000000000000000, -1.836970198721030181E-16, -2.465190328815661892E-32 ) ) ;
#3399=CARTESIAN_POINT ( 'NONE',  ( 200.0000000000000000, 5.800536564436440834, 18.10358378745109320 ) ) ;
#3413=CARTESIAN_POINT ( 'NONE',  ( -259.2033419157646676, -6.730120644403663199, 6.730120644403451813 ) ) ;
#3422=CARTESIAN_POINT ( 'NONE',  ( 199.9999999999999147, -15.08385563027219156, -11.56407354529143205 ) ) ;
#3426=CARTESIAN_POINT ( 'NONE',  ( 199.0066333181452478, 19.18530965003537858, -5.635992787424102701 ) ) ;
#3459=CARTESIAN_POINT ( 'NONE',  ( 200.0000000000000853, -13.44239485489230290, 13.44239485489200803 ) ) ;
#3504=CARTESIAN_POINT ( 'NONE',  ( 200.0000000000001705, -16.91021041590709473, -8.683373960011902426 ) ) ;
#3528=CARTESIAN_POINT ( 'NONE',  ( 200.0000000000000284, 12.51656570147539327, 14.30544205704861760 ) ) ;
#3541=CARTESIAN_POINT ( 'NONE',  ( -91.56559293963834989, -16.03295912088728414, 16.03295912088688269 ) ) ;
#3553=CARTESIAN_POINT ( 'NONE',  ( 200.0000000000002274, -18.85575486854367355, -2.482946933799725642 ) ) ;
#3556=CARTESIAN_POINT ( 'NONE',  ( 199.0060750228415429, 7.941611777091910795, -18.35102805502410561 ) ) ;
#3574=CARTESIAN_POINT ( 'NONE',  ( 151.7948205124836250, -23.49921654116371883, 23.49921654116317526 ) ) ;
#3583=CARTESIAN_POINT ( 'NONE',  ( -280.0000000000000000, -10.00000000000005151, -6.902532920683853297E-30 ) ) ;
#3585=CARTESIAN_POINT ( 'NONE',  ( 200.0000000000005684, -1.253076495463282924, 18.97792690268338234 ) ) ;
#3590=CARTESIAN_POINT ( 'NONE',  ( -30.26275506840324070, 1.198031551616724366, -57.76657404653984429 ) ) ;
#3618=CARTESIAN_POINT ( 'NONE',  ( 199.0253302299943812, -18.92118621875344786, 6.501515187515664707 ) ) ;
#3632=CARTESIAN_POINT ( 'NONE',  ( 200.0000000000000853, -13.44239485489230290, 13.44239485489200803 ) ) ;
#3648=CARTESIAN_POINT ( 'NONE',  ( 146.6084372240433993, -24.48358557860353457, 24.48358557860296258 ) ) ;
#3662=CARTESIAN_POINT ( 'NONE',  ( 199.9999999999998579, -4.480715147297966716, 18.47471730767352938 ) ) ;
#3663=CARTESIAN_POINT ( 'NONE',  ( 199.9999999999999716, -14.29283438936585604, -12.53096660533077689 ) ) ;
#3675=CARTESIAN_POINT ( 'NONE',  ( 14.38125909742180220, 39.01709431150892016, 17.55144818341517166 ) ) ;
#3678=CARTESIAN_POINT ( 'NONE',  ( -280.0000000000000000, -14.14213562373118549, 14.14213562373078936 ) ) ;
#3693=CARTESIAN_POINT ( 'NONE',  ( 199.0058097323984327, 9.278912463403225175, -17.71230630396810213 ) ) ;
#3724=CARTESIAN_POINT ( 'NONE',  ( 199.9999999999998863, 18.69362872516077800, 3.425107952296777114 ) ) ;
#3730=CARTESIAN_POINT ( 'NONE',  ( 57.59792236341147031, 26.56190807104720975, -26.56190807104655249 ) ) ;
#3755=CARTESIAN_POINT ( 'NONE',  ( 199.9999999999999716, 18.51141176942600097, 4.336711825884415283 ) ) ;
#3761=CARTESIAN_POINT ( 'NONE',  ( 199.0074854128475579, 2.768696461275208520, -19.80384161416936806 ) ) ;
#3766=CARTESIAN_POINT ( 'NONE',  ( -135.8532207217289738, 21.81201906317798134, -21.81201906317747685 ) ) ;
#3768=CARTESIAN_POINT ( 'NONE',  ( 200.0000000000001705, -18.10265802883496278, 5.810802590798905598 ) ) ;
#3771=CARTESIAN_POINT ( 'NONE',  ( 199.0206025836015442, 6.413712542583970944, 18.94893284924772203 ) ) ;
#3802=CARTESIAN_POINT ( 'NONE',  ( 199.9999999999999716, 18.70067531203203970, -3.379044910449504169 ) ) ;
#3803=CARTESIAN_POINT ( 'NONE',  ( 200.0000000000000000, -13.65901895451712811, -13.21854774209566585 ) ) ;
#3814=CARTESIAN_POINT ( 'NONE',  ( 199.0150730930814689, 15.28768747664870453, 12.90128171110900013 ) ) ;
#3816=CARTESIAN_POINT ( 'NONE',  ( -105.3755690713226585, 41.18208027870575449, 15.38646221621837107 ) ) ;
#3829=CARTESIAN_POINT ( 'NONE',  ( 199.9999999999999716, -18.76480772196043034, -3.095184993347289026 ) ) ;
#3832=CARTESIAN_POINT ( 'NONE',  ( 199.0093721751683518, -2.288394243462712030, -19.86801947894618792 ) ) ;
#3860=CARTESIAN_POINT ( 'NONE',  ( 200.0000000000000568, 5.208214048020466613, 18.28294570233482119 ) ) ;
#3868=CARTESIAN_POINT ( 'NONE',  ( -238.4067589809705794, 0.6820004458491113475, -57.25054294077229144 ) ) ;
#3869=CARTESIAN_POINT ( 'NONE',  ( 199.0251223662492635, -5.665586242881555101, 19.18612710904600149 ) ) ;
#3888=ORIENTED_EDGE ( 'NONE', *, *, #19870, .T. ) ;
#3899=CARTESIAN_POINT ( 'NONE',  ( 199.9999999999999716, 18.84369875136934880, -2.460375794728051790 ) ) ;
#3906=CARTESIAN_POINT ( 'NONE',  ( 199.0059208051008852, 8.690306674284110855, -18.00847358856242408 ) ) ;
#3915=CARTESIAN_POINT ( 'NONE',  ( 199.0173417939125784, 12.16728005963107329, 15.88742495833056800 ) ) ;
#3941=CARTESIAN_POINT ( 'NONE',  ( 199.9999999999999432, 18.93973332185608172, 1.567235916626209535 ) ) ;
#3942=CARTESIAN_POINT ( 'NONE',  ( 199.9999999999999716, -16.61824216245382502, -9.229554904678261451 ) ) ;
#3951=CARTESIAN_POINT ( 'NONE',  ( 199.0221514193071926, 3.032938341077176414, 19.78261031040590012 ) ) ;
#3952=CARTESIAN_POINT ( 'NONE',  ( 4.995406935893290878, 39.06748935135239265, -39.06748935135144762 ) ) ;
#3966=CARTESIAN_POINT ( 'NONE',  ( 199.9999999999998579, -18.00099009291985297, -6.105420735363839668 ) ) ;
#3971=CARTESIAN_POINT ( 'NONE',  ( 199.0198127172867828, -18.35326955327933618, -7.958687714023728432 ) ) ;
#3997=CARTESIAN_POINT ( 'NONE',  ( 199.9999999999998579, 13.86282612285610938, 13.00154682524819805 ) ) ;
#4003=CARTESIAN_POINT ( 'NONE',  ( -86.96347745069644475, -15.38646221621738164, -41.18208027870615240 ) ) ;
#4004=CARTESIAN_POINT ( 'NONE',  ( 199.0220573263155188, 3.250837537642027542, 19.73775173755759127 ) ) ;
#4031=CARTESIAN_POINT ( 'NONE',  ( 199.9999999999999147, 15.61914218176268143, 10.83067004454828641 ) ) ;
#4038=CARTESIAN_POINT ( 'NONE',  ( 199.0065087001378572, 6.107362818253672998, -19.04251412529381327 ) ) ;
#4046=CARTESIAN_POINT ( 'NONE',  ( 199.0161420530203600, 13.89456085230456850, 14.38651294782529888 ) ) ;
#4073=CARTESIAN_POINT ( 'NONE',  ( 200.0000000000000853, 16.14603016630555743, -10.01676266068942667 ) ) ;
#4074=CARTESIAN_POINT ( 'NONE',  ( 199.9999999999998863, -17.79060443684709369, -6.693342262146931176 ) ) ;
#4078=DIRECTION ( 'NONE',  ( 0.000000000000000000, -0.7071067811865561215, 0.7071067811865389130 ) ) ;
#4084=CARTESIAN_POINT ( 'NONE',  ( 199.0206793870229376, 6.297627498482031072, 19.03991857512456320 ) ) ;
#4085=CARTESIAN_POINT ( 'NONE',  ( 14.38125909742181108, 39.01709431150961649, -39.01709431150867147 ) ) ;
#4088=CARTESIAN_POINT ( 'NONE',  ( 19.06497207195979726, 38.31983398719604139, 18.24870850772803976 ) ) ;
#4098=CARTESIAN_POINT ( 'NONE',  ( 200.0000000000000853, -13.44239485489230290, 13.44239485489200803 ) ) ;
#4101=CARTESIAN_POINT ( 'NONE',  ( 199.0111317961331281, -6.131174403448985011, -19.03732645848564431 ) ) ;
#4135=CARTESIAN_POINT ( 'NONE',  ( 199.9999999999998863, 12.28125103214278901, 14.50804496155330447 ) ) ;
#4143=CARTESIAN_POINT ( 'NONE',  ( -280.0000000000000000, 14.14213562373108246, -14.14213562373078581 ) ) ;
#4144=CARTESIAN_POINT ( 'NONE',  ( 199.0262541782678340, -11.79586192385960430, 16.15815307234555576 ) ) ;
#4169=CARTESIAN_POINT ( 'NONE',  ( 199.9999999999999716, 16.82248425547956217, 8.841323171526189739 ) ) ;
#4175=CARTESIAN_POINT ( 'NONE',  ( 199.0087111817176435, -0.6649071253763039202, -19.99597453042600392 ) ) ;
#4180=CARTESIAN_POINT ( 'NONE',  ( 200.0000000000000284, -14.89458464808834748, 11.81399803044240038 ) ) ;
#4183=CARTESIAN_POINT ( 'NONE',  ( 199.0152755141893692, 15.03153897770602221, 13.19647528785794677 ) ) ;
#4209=CARTESIAN_POINT ( 'NONE',  ( 200.0000000000001421, 16.60215271479902910, 9.252637072649047667 ) ) ;
#4211=CARTESIAN_POINT ( 'NONE',  ( 199.9999999999999147, -17.31672820518381783, 7.849270303112303004 ) ) ;
#4221=CARTESIAN_POINT ( 'NONE',  ( 199.0168430542531155, 12.91005451537445126, 15.29445721284177573 ) ) ;
#4224=CARTESIAN_POINT ( 'NONE',  ( -192.9588430854690273, 10.23066800229588758, -66.79921049721882298 ) ) ;
#4226=CARTESIAN_POINT ( 'NONE',  ( 136.1360204305621551, 31.79587985999232558, 24.77266263493161702 ) ) ;
#4239=CARTESIAN_POINT ( 'NONE',  ( 199.0181825105790665, -16.81808889125263207, -10.83063377519274795 ) ) ;
#4266=CARTESIAN_POINT ( 'NONE',  ( 199.9999999999998863, 17.10417011681778732, 8.282922153951966848 ) ) ;
#4272=CARTESIAN_POINT ( 'NONE',  ( 0.2972598230769990524, -18.14793986248671231, -38.42060263243687501 ) ) ;
#4273=CARTESIAN_POINT ( 'NONE',  ( 199.0263771353516233, -14.14574067859894413, 14.14574067859863682 ) ) ;
#4289=CARTESIAN_POINT ( 'NONE',  ( -208.1127848780265026, 10.60833733269551615, -10.60833733269529766 ) ) ;
#4301=CARTESIAN_POINT ( 'NONE',  ( 200.0000000000000000, 6.097653648161206696, 18.01359495397503352 ) ) ;
#4308=CARTESIAN_POINT ( 'NONE',  ( 199.0137359473271488, -10.84478214295758036, -16.80398351328055639 ) ) ;
#4317=CARTESIAN_POINT ( 'NONE',  ( 199.0145894300637792, 15.86095929198710586, 12.18642508278280623 ) ) ;
#4340=CARTESIAN_POINT ( 'NONE',  ( 199.9999999999998863, -5.231270638550959085, -18.27112563740264761 ) ) ;
#4341=CARTESIAN_POINT ( 'NONE',  ( 199.9999999999999716, 9.498725063112413380, -16.45837312633763005 ) ) ;
#4350=CARTESIAN_POINT ( 'NONE',  ( 199.0255859347418834, -7.628281087858428400, 18.49319637005222816 ) ) ;
#4351=CARTESIAN_POINT ( 'NONE',  ( -280.0000000000000568, -14.14213562373049449, -42.42640687119305198 ) ) ;
#4353=CARTESIAN_POINT ( 'NONE',  ( 184.8905102610680444, 41.77492675555983936, 14.79361573936436081 ) ) ;
#4368=CARTESIAN_POINT ( 'NONE',  ( 199.0152737994447136, -13.19951906643276374, -15.03942049639883294 ) ) ;
#4384=B_SPLINE_CURVE_WITH_KNOTS ( 'NONE', 3,
 ( #21596, #15590, #25478, #17850, #1508, #15345, #5496, #9483, #3766, #17719, #19463, #17587, #19594, #7605, #15719, #17464, #13863, #21856, #19856, #11737, #1642, #26000, #1251, #23978, #9355, #25607, #7350, #15463, #23590, #5369 ),
 .UNSPECIFIED., .F., .F.,
 ( 4, 2, 2, 2, 2, 2, 2, 2, 2, 2, 2, 2, 2, 2, 4 ),
 ( 0.000000000000000000, 0.1357259735107005372, 0.1651108541090157700, 0.1944957347073310028, 0.3598804999793158710, 0.3867117631979620773, 0.4135430264166082281, 0.5789277916885930964, 0.6062785021374117456, 0.6336292125862302838, 0.8508620842112317728, 0.8814014469398914198, 0.9119408096685510667, 0.9559704048342755334, 0.9980677081714144361 ),
 .UNSPECIFIED. ) ;
#4394=CARTESIAN_POINT ( 'NONE',  ( 199.9999999999998579, 18.23094931701148269, -5.355502299499542040 ) ) ;
#4399=CARTESIAN_POINT ( 'NONE',  ( 184.8905102610680444, -14.79361573936399665, 14.79361573936367158 ) ) ;
#4400=CARTESIAN_POINT ( 'NONE',  ( 199.0242446922718784, -2.616032970993653173, 19.83497009005848710 ) ) ;
#4413=CARTESIAN_POINT ( 'NONE',  ( -135.8532207217289738, -6.472252184284280396, 6.472252184284099208 ) ) ;
#4424=CARTESIAN_POINT ( 'NONE',  ( 200.0000000000000284, 4.307699855108636733, 18.51410484079663377 ) ) ;
#4430=CARTESIAN_POINT ( 'NONE',  ( 199.0232879746372134, -20.00360196692749071, -0.1645009869758431997 ) ) ;
#4440=CARTESIAN_POINT ( 'NONE',  ( 199.0089741461167989, 19.95552976068599804, 1.321036586804004820 ) ) ;
#4448=DIRECTION ( 'NONE',  ( -1.000000000000000000, -1.836970198721030181E-16, -2.465190328815661892E-32 ) ) ;
#4456=CARTESIAN_POINT ( 'NONE',  ( 199.0061375790170644, 7.656915158548016187, -18.47094169875700942 ) ) ;
#4467=CARTESIAN_POINT ( 'NONE',  ( 199.9999999999999147, -6.121038220875967717, -17.99280653461927315 ) ) ;
#4470=FACE_BOUND ( 'NONE', #8196, .T. ) ;
#4476=CARTESIAN_POINT ( 'NONE',  ( 199.0117673552712745, 18.58883966351390526, 7.374690901580303937 ) ) ;
#4477=CARTESIAN_POINT ( 'NONE',  ( 199.9999999999999432, 14.14213562373110911, -14.14213562373072364 ) ) ;
#4480=CARTESIAN_POINT ( 'NONE',  ( 4.995406935893283773, 39.06748935135171052, 17.50105314357239195 ) ) ;
#4493=CARTESIAN_POINT ( 'NONE',  ( 199.0223302282441296, -19.84245377806801613, -2.613091800807908260 ) ) ;
#4527=CARTESIAN_POINT ( 'NONE',  ( 200.0000000000001137, 15.89309473284322749, -10.41337480477382371 ) ) ;
#4528=CLOSED_SHELL ( 'NONE', ( #22740, #10620, #25086, #15305, #15945, #11187, #4861, #24012, #4918 ) ) ;
#4531=CARTESIAN_POINT ( 'NONE',  ( 130.8568914410475088, -52.36146031193413108, -4.207082182990267150 ) ) ;
#4532=CARTESIAN_POINT ( 'NONE',  ( 199.0093797572272081, 19.86600527971208763, 2.306481033292959726 ) ) ;
#4561=CARTESIAN_POINT ( 'NONE',  ( 200.0000000000000000, -11.82748140626729239, 14.88626897493814027 ) ) ;
#4567=CARTESIAN_POINT ( 'NONE',  ( 199.0207495982873809, -19.04631292825652622, -6.112231798784620196 ) ) ;
#4577=CARTESIAN_POINT ( 'NONE',  ( 199.0066333181452478, 19.18530965003537858, -5.635992787424102701 ) ) ;
#4591=CARTESIAN_POINT ( 'NONE',  ( 199.0067109444755147, 5.297717337603594423, -19.32538706503994064 ) ) ;
#4603=CARTESIAN_POINT ( 'NONE',  ( 200.0000000000000853, 11.56430744387933274, -15.08818561847743922 ) ) ;
#4614=CARTESIAN_POINT ( 'NONE',  ( 199.0061394614210144, 18.47445098178025447, -7.648446613688572704 ) ) ;
#4615=CARTESIAN_POINT ( 'NONE',  ( 151.7948205124836534, -51.78348778862529400, -4.785054706299085581 ) ) ;
#4628=CARTESIAN_POINT ( 'NONE',  ( 199.0236444319429268, -19.98745889671670284, 0.8241971460415670192 ) ) ;
#4656=CARTESIAN_POINT ( 'NONE',  ( 199.9999999999997442, 8.817246258963736594, -16.83121203733840332 ) ) ;
#4660=CARTESIAN_POINT ( 'NONE',  ( -135.8532207217289738, -6.472252184284280396, 6.472252184284099208 ) ) ;
#4661=CARTESIAN_POINT ( 'NONE',  ( 199.0130717410369812, 17.47129959974107294, 9.736724163761770967 ) ) ;
#4676=CARTESIAN_POINT ( 'NONE',  ( 199.0262541782678340, -11.79586192385960430, 16.15815307234555576 ) ) ;
#4696=CARTESIAN_POINT ( 'NONE',  ( 199.0173355507466226, -15.87315179554041045, -12.16952887920782445 ) ) ;
#4710=CARTESIAN_POINT ( 'NONE',  ( 199.0116003924211725, 18.71458825927322422, 7.055789865482638312 ) ) ;
#4733=CARTESIAN_POINT ( 'NONE',  ( 200.0000000000002842, 11.06692676694369304, -15.45668394874709506 ) ) ;
#4734=CARTESIAN_POINT ( 'NONE',  ( 199.9999999999999716, -3.099454106775636930, -18.75032367107563758 ) ) ;
#4746=CARTESIAN_POINT ( 'NONE',  ( 199.0089039147429446, 19.99546107379537929, 1.174471671411769780 ) ) ;
#4747=CARTESIAN_POINT ( 'NONE',  ( 130.8568914410475088, -24.07718906446864793, -32.49135343045505664 ) ) ;
#4763=CARTESIAN_POINT ( 'NONE',  ( 199.0232268534825835, -20.00153578626446915, -0.3291254421221458948 ) ) ;
#4794=CARTESIAN_POINT ( 'NONE',  ( 200.0000000000002274, 18.09557305485218848, -5.802546270622393365 ) ) ;
#4799=CARTESIAN_POINT ( 'NONE',  ( 199.0163148259956358, 13.65645126726637670, 14.61284818176725331 ) ) ;
#4829=CARTESIAN_POINT ( 'NONE',  ( 199.0156165598358768, -13.68207045034666969, -14.60203791353019476 ) ) ;
#4840=CARTESIAN_POINT ( 'NONE',  ( 199.0120006491917479, 18.40818734026414560, 7.815811290271758693 ) ) ;
#4861=ADVANCED_FACE ( 'NONE', ( #11834 ), #1736, .F. ) ;
#4867=CARTESIAN_POINT ( 'NONE',  ( 200.0000000000001705, 1.541304384858841692, -18.93928971938424155 ) ) ;
#4868=CARTESIAN_POINT ( 'NONE',  ( 199.9999999999999716, -6.703600881535439093, -17.78416426705615550 ) ) ;
#4877=CARTESIAN_POINT ( 'NONE',  ( 199.0053211798077086, 14.13837298227953987, -14.13837298578013701 ) ) ;
#4878=CARTESIAN_POINT ( 'NONE',  ( 19.06497207195980792, 10.03556273973447155, -10.03556273973422286 ) ) ;
#4891=CARTESIAN_POINT ( 'NONE',  ( 199.0263095778509808, -15.67393427090936875, 12.43211889955359162 ) ) ;
#4916=CARTESIAN_POINT ( 'NONE',  ( 199.9999999999998863, 12.98615309696526587, -13.88358464575571283 ) ) ;
#4918=ADVANCED_FACE ( 'NONE', ( #16621 ), #17409, .T. ) ;
#4921=CARTESIAN_POINT ( 'NONE',  ( 199.0125740919301336, 17.92725630381683644, 8.864156431172764528 ) ) ;
#4943=CARTESIAN_POINT ( 'NONE',  ( 163.1118516004056573, -19.27778845538787422, 19.27778845538743724 ) ) ;
#4955=CARTESIAN_POINT ( 'NONE',  ( 199.9999999999999432, -10.30972604295016559, 15.97265043433685250 ) ) ;
#4959=CARTESIAN_POINT ( 'NONE',  ( 199.0250768083106436, -19.24006491846622069, 5.486913247009519878 ) ) ;
#4972=CARTESIAN_POINT ( 'NONE',  ( 199.0055651108938832, 16.81514173603054374, -10.81990435933588302 ) ) ;
#4989=CARTESIAN_POINT ( 'NONE',  ( 199.0117626354723370, -7.365673525892063367, -18.59241149604612886 ) ) ;
#4999=CARTESIAN_POINT ( 'NONE',  ( 200.0000000000000284, -15.63511319855579629, -10.80754414709790190 ) ) ;
#5008=CARTESIAN_POINT ( 'NONE',  ( 199.0061264496102353, 18.45002901997423095, -7.707159767720078491 ) ) ;
#5009=CARTESIAN_POINT ( 'NONE',  ( 146.6084372240433709, -52.76785682606510619, -3.800685668859292043 ) ) ;
#5023=CARTESIAN_POINT ( 'NONE',  ( 199.0227232939661519, -19.93874224789216143, -1.638880401382246443 ) ) ;
#5048=CARTESIAN_POINT ( 'NONE',  ( 199.9999999999998863, -2.943496653232010374, -18.77345647985907462 ) ) ;
#5053=CARTESIAN_POINT ( 'NONE',  ( 199.0196638708318631, 8.237985373594881366, 18.22956011771260165 ) ) ;
#5066=CARTESIAN_POINT ( 'NONE',  ( 199.0257180514102799, -8.261434504147922908, 18.22213678534573589 ) ) ;
#5068=CARTESIAN_POINT ( 'NONE',  ( -192.9588430854690273, 66.79921049724377724, -10.23066800231904239 ) ) ;
#5085=CARTESIAN_POINT ( 'NONE',  ( 199.9999999999998579, 3.088973468740698447, 18.75625871509165776 ) ) ;
#5114=CARTESIAN_POINT ( 'NONE',  ( 199.0199587825621563, -18.46922402431326304, -7.678974719652290837 ) ) ;
#5126=CARTESIAN_POINT ( 'NONE',  ( 199.9999999999999716, -9.233471789954972309, -16.61280101608961246 ) ) ;
#5136=CARTESIAN_POINT ( 'NONE',  ( -86.96347745069644475, -43.67073346367964604, -12.89780903124457545 ) ) ;
#5150=CARTESIAN_POINT ( 'NONE',  ( 199.9999999999997726, -5.383989893674753446, 18.23209102328170061 ) ) ;
#5176=CARTESIAN_POINT ( 'NONE',  ( 199.9999999999998863, -4.016713260438497635, -18.57371263647062420 ) ) ;
#5179=CARTESIAN_POINT ( 'NONE',  ( 199.0068072339493597, 19.36029496603142874, -5.002335373038918398 ) ) ;
#5198=( NAMED_UNIT ( * ) SI_UNIT ( $, .STERADIAN. ) SOLID_ANGLE_UNIT ( ) );
#5207=CARTESIAN_POINT ( 'NONE',  ( 199.0263095778509808, -15.67393427090936875, 12.43211889955359162 ) ) ;
#5212=CARTESIAN_POINT ( 'NONE',  ( -265.0000000000000000, -4.867971026610730343E-14, -6.532754371361504014E-30 ) ) ;
#5234=CARTESIAN_POINT ( 'NONE',  ( 199.0199679947243112, -18.47654620739217890, -7.661348058496780133 ) ) ;
#5244=CARTESIAN_POINT ( 'NONE',  ( 199.9999999999998863, -9.504749071264818383, -16.45922038047892144 ) ) ;
#5255=EDGE_CURVE ( 'NONE', #5806, #122, #9587, .T. ) ;
#5270=CARTESIAN_POINT ( 'NONE',  ( 199.9999999999999147, -8.688421465551046552, 16.91138275242808575 ) ) ;
#5293=CARTESIAN_POINT ( 'NONE',  ( 199.9999999999999147, -15.17855064416508526, -11.43956010876637563 ) ) ;
#5296=CARTESIAN_POINT ( 'NONE',  ( 199.0054082256929746, 12.16974446990029790, -15.87805152391047159 ) ) ;
#5314=CARTESIAN_POINT ( 'NONE',  ( -213.1075012329537230, 9.698598906450543566, -9.698598906450348167 ) ) ;
#5324=CARTESIAN_POINT ( 'NONE',  ( 199.0263356842403653, -15.36141226383640301, 12.81629321302553848 ) ) ;
#5335=FACE_OUTER_BOUND ( 'NONE', #21939, .T. ) ;
#5359=CARTESIAN_POINT ( 'NONE',  ( 199.0233250129033991, -20.00353002365851651, -0.06339277442724530753 ) ) ;
#5369=CARTESIAN_POINT ( 'NONE',  ( 199.0053211798077086, 14.13837298227953987, -14.13837298578013701 ) ) ;
#5371=CARTESIAN_POINT ( 'NONE',  ( 199.9999999999996874, -18.99916535394237727, -0.6249076428296399532 ) ) ;
#5399=CARTESIAN_POINT ( 'NONE',  ( 199.0053211801402142, 14.13668625429389891, -14.14005970859717642 ) ) ;
#5400=CARTESIAN_POINT ( 'NONE',  ( 199.9999999999995737, 11.06459441337805494, 15.46579378046570952 ) ) ;
#5413=CARTESIAN_POINT ( 'NONE',  ( -91.56559293963834989, -16.03295912088728414, 16.03295912088688269 ) ) ;
#5423=CARTESIAN_POINT ( 'NONE',  ( 199.9999999999999147, -13.65919145721374761, -13.21838778087559518 ) ) ;
#5427=CARTESIAN_POINT ( 'NONE',  ( 199.0058938177734547, 17.94521767341456098, -8.824629201450257199 ) ) ;
#5447=CARTESIAN_POINT ( 'NONE',  ( 14.38125909742180752, 10.73282306404735387, -10.73282306404708919 ) ) ;
#5454=VERTEX_POINT ( 'NONE', #17823 ) ;
#5455=ORIENTED_EDGE ( 'NONE', *, *, #14107, .T. ) ;
#5457=CARTESIAN_POINT ( 'NONE',  ( 199.0263771350486763, -14.37646237564524476, 13.91501816527019919 ) ) ;
#5471=AXIS2_PLACEMENT_3D ( 'NONE', #23943, #7196, #15433 ) ;
#5486=CARTESIAN_POINT ( 'NONE',  ( 199.0263117864500657, -15.86583567901655911, 12.25628060790395679 ) ) ;
#5496=CARTESIAN_POINT ( 'NONE',  ( -192.9588430854689989, 38.51493924976983152, -38.51493924976893624 ) ) ;
#5498=CARTESIAN_POINT ( 'NONE',  ( 200.0000000000001137, -16.46591192518303970, -9.498466322123544359 ) ) ;
#5510=CARTESIAN_POINT ( 'NONE',  ( 163.1118516004056573, -19.27778845538787422, 19.27778845538743724 ) ) ;
#5514=ORIENTED_EDGE ( 'NONE', *, *, #17819, .T. ) ;
#5522=DIRECTION ( 'NONE',  ( -1.000000000000000000, -1.836970198721030181E-16, -1.232595164407830946E-32 ) ) ;
#5523=CARTESIAN_POINT ( 'NONE',  ( 199.9999999999998295, 10.02997355460652429, 16.14748021227288532 ) ) ;
#5536=CARTESIAN_POINT ( 'NONE',  ( -105.3755690713226585, 12.89780903124349720, 43.67073346367994446 ) ) ;
#5539=CARTESIAN_POINT ( 'NONE',  ( 199.9999999999999432, -14.14213562373115884, 14.14213562373085153 ) ) ;
#5548=CARTESIAN_POINT ( 'NONE',  ( 199.9999999999999716, -6.704437273156823807, -17.78382994799445527 ) ) ;
#5551=CARTESIAN_POINT ( 'NONE',  ( 199.0056007646616933, 10.55815519723130969, -16.98307562551513072 ) ) ;
#5584=CARTESIAN_POINT ( 'NONE',  ( 200.0000000000000284, -9.508146755684434126, 16.46234680784547777 ) ) ;
#5590=CARTESIAN_POINT ( 'NONE',  ( -162.0762913951020892, 1.198031840456041497, -57.76657433537918251 ) ) ;
#5615=CARTESIAN_POINT ( 'NONE',  ( 200.0000000000000000, 16.22959744068430155, -9.888235504304919488 ) ) ;
#5616=CARTESIAN_POINT ( 'NONE',  ( 199.0221430437530898, -19.77959184285664307, -3.052687890358243283 ) ) ;
#5623=CARTESIAN_POINT ( 'NONE',  ( 199.0053211804427633, 14.13331159297750617, -14.14343255912447361 ) ) ;
#5626=CARTESIAN_POINT ( 'NONE',  ( 200.0000000000002274, -14.59760583945227808, 12.17906594671359244 ) ) ;
#5652=CARTESIAN_POINT ( 'NONE',  ( 200.0000000000001990, -4.022463818607304731, 18.57981244883409744 ) ) ;
#5665=CARTESIAN_POINT ( 'NONE',  ( -86.96347745069644475, 41.18208027870576871, 15.38646221621837107 ) ) ;
#5668=CARTESIAN_POINT ( 'NONE',  ( 4.995406935893289102, 10.78321810389013002, -10.78321810388986712 ) ) ;
#5677=CARTESIAN_POINT ( 'NONE',  ( 200.0000000000000568, -17.44062545528135999, -7.562669404541021656 ) ) ;
#5681=CARTESIAN_POINT ( 'NONE',  ( 199.0062801269303350, 18.72091001596172433, -7.031396878026334285 ) ) ;
#5710=CARTESIAN_POINT ( 'NONE',  ( 199.9999999999999716, 18.09021486607068496, 5.826594753398616433 ) ) ;
#5717=CARTESIAN_POINT ( 'NONE',  ( 184.8905102610680444, 13.49065550809826952, -13.49065550809790359 ) ) ;
#5744=CARTESIAN_POINT ( 'NONE',  ( 199.9999999999999432, 18.09516392985831601, -5.803866375870236460 ) ) ;
#5757=CARTESIAN_POINT ( 'NONE',  ( 200.0000000000000568, -15.63904601878861733, 10.81246610429574595 ) ) ;
#5760=CARTESIAN_POINT ( 'NONE',  ( 199.0140795438509826, 16.43701665320993044, 11.39707250661459348 ) ) ;
#5788=CARTESIAN_POINT ( 'NONE',  ( 199.9999999999999147, 19.00141375156598045, 0.3223421948013435179 ) ) ;
#5789=CARTESIAN_POINT ( 'NONE',  ( 199.9999999999999432, -18.37296950073040236, 4.918342949125168673 ) ) ;
#5800=CARTESIAN_POINT ( 'NONE',  ( 199.0233480856092001, 0.0005622888856919192003, 20.00362916157371629 ) ) ;
#5801=CARTESIAN_POINT ( 'NONE',  ( 91.82158438592158234, -12.16597498397778843, 12.16597498397750954 ) ) ;
#5804=CARTESIAN_POINT ( 'NONE',  ( -162.0762913951020892, 1.198031840385732849, -1.198031840385733515 ) ) ;
#5806=VERTEX_POINT ( 'NONE', #12297 ) ;
#5816=CARTESIAN_POINT ( 'NONE',  ( 200.0000000000000853, -18.58433719308212773, 4.010382776060092525 ) ) ;
#5821=CARTESIAN_POINT ( 'NONE',  ( 199.0163032586025622, -14.59919991228128922, -13.67396374720910757 ) ) ;
#5848=CARTESIAN_POINT ( 'NONE',  ( 199.9999999999999432, 16.89472078740815775, 8.702431973737679627 ) ) ;
#5854=CARTESIAN_POINT ( 'NONE',  ( 151.7948205124836534, -23.49921654115981084, -33.06932595376387951 ) ) ;
#5881=CARTESIAN_POINT ( 'NONE',  ( 199.9999999999999716, 18.70042687752384936, -3.380346622114776434 ) ) ;
#5887=CARTESIAN_POINT ( 'NONE',  ( 199.0093721751683518, -2.288394243462712030, -19.86801947894618792 ) ) ;
#5896=CARTESIAN_POINT ( 'NONE',  ( 199.0198237862232133, 7.937771492746675150, 18.36232769351375538 ) ) ;
#5926=CARTESIAN_POINT ( 'NONE',  ( 200.0000000000000000, 17.99290950227088004, 6.120759354987654000 ) ) ;
#5927=CARTESIAN_POINT ( 'NONE',  ( 199.9999999999999147, -17.05647522489845969, -8.409730364717644235 ) ) ;
#5936=CARTESIAN_POINT ( 'NONE',  ( 199.0195099801769061, 8.518539848973487594, 18.09882726175286649 ) ) ;
#5937=CARTESIAN_POINT ( 'NONE',  ( 130.8568914410475372, 4.207082182992923691, -4.207082182992794017 ) ) ;
#5939=CARTESIAN_POINT ( 'NONE',  ( 0.2972598230769938343, 10.13633138497486286, -10.13633138497461594 ) ) ;
#5950=CARTESIAN_POINT ( 'NONE',  ( 199.9999999999999432, -17.61942792365240607, -7.131405496535110800 ) ) ;
#5954=CARTESIAN_POINT ( 'NONE',  ( 199.0156165598358768, -13.68207045034666969, -14.60203791353019476 ) ) ;
#5982=CARTESIAN_POINT ( 'NONE',  ( 199.9999999999998863, 6.967860089407453827, 17.68684069956508154 ) ) ;
#5989=CARTESIAN_POINT ( 'NONE',  ( -135.8532207217289738, -6.472252184283586729, -50.09629031063973770 ) ) ;
#5990=CARTESIAN_POINT ( 'NONE',  ( 199.0223319294094892, 2.599958516019920118, 19.83413122362564351 ) ) ;
#6018=CARTESIAN_POINT ( 'NONE',  ( 199.9999999999999432, 18.08994308216479752, 5.827519331295367699 ) ) ;
#6025=CARTESIAN_POINT ( 'NONE',  ( 199.0138211924391385, -10.98290011267725141, -16.71408225681557980 ) ) ;
#6034=CARTESIAN_POINT ( 'NONE',  ( 199.0194208361885444, 8.684746017668368623, 18.01861981654000999 ) ) ;
#6060=CARTESIAN_POINT ( 'NONE',  ( 200.0000000000000000, 16.44874601624584187, 9.522804452304930223 ) ) ;
#6063=CARTESIAN_POINT ( 'NONE',  ( 200.0000000000000000, -13.87499997850619060, -12.99183991311445929 ) ) ;
#6072=CARTESIAN_POINT ( 'NONE',  ( 199.0230791219081254, 0.7206054984853534906, 19.99107781132848416 ) ) ;
#6073=CARTESIAN_POINT ( 'NONE',  ( 19.06497207195981147, 38.31983398719673772, -38.31983398719579981 ) ) ;
#6075=CARTESIAN_POINT ( 'NONE',  ( 14.38125909742180220, 39.01709431150892016, 17.55144818341517166 ) ) ;
#6084=CARTESIAN_POINT ( 'NONE',  ( 199.9999999999999147, -17.05087848619496782, 8.411269650559694000 ) ) ;
#6087=CARTESIAN_POINT ( 'NONE',  ( 199.0097900131551114, -3.258944298918965199, -19.73026277452668609 ) ) ;
#6113=CARTESIAN_POINT ( 'NONE',  ( 200.0000000000000000, 9.224923989862913842, 16.61864493261536424 ) ) ;
#6119=CARTESIAN_POINT ( 'NONE',  ( -259.2033419157646676, -35.01439189186523748, -21.55415060305881170 ) ) ;
#6120=CARTESIAN_POINT ( 'NONE',  ( 199.0253172846266523, -6.444568167316012008, 18.94088585829734228 ) ) ;
#6144=CARTESIAN_POINT ( 'NONE',  ( 200.0000000000000000, 16.89533303742294734, 8.701242830477832868 ) ) ;
#6151=CARTESIAN_POINT ( 'NONE',  ( 199.0056007646616933, 10.55815519723130969, -16.98307562551513072 ) ) ;
#6153=EDGE_CURVE ( 'NONE', #17548, #20820, #8576, .T. ) ;
#6161=CARTESIAN_POINT ( 'NONE',  ( 199.0190933210857906, 9.274233341078666371, 17.72222919763310856 ) ) ;
#6184=CARTESIAN_POINT ( 'NONE',  ( 199.9999999999998863, 18.69362872516077800, 3.425107952296777114 ) ) ;
#6185=CARTESIAN_POINT ( 'NONE',  ( 200.0000000000000284, -18.85585617391987867, -2.482101612725928330 ) ) ;
#6196=CARTESIAN_POINT ( 'NONE',  ( 199.0255894194985729, -7.644541030299115469, 18.48648443203342140 ) ) ;
#6198=CARTESIAN_POINT ( 'NONE',  ( -213.1075012329537230, 9.698598906438871126, -66.26714140136179765 ) ) ;
#6200=CARTESIAN_POINT ( 'NONE',  ( 91.82158438592158234, 44.40256751092319121, 12.16597498400105515 ) ) ;
#6209=CIRCLE ( 'NONE', #705, 10.00000000000000000 ) ;
#6212=CARTESIAN_POINT ( 'NONE',  ( 199.9999999999998579, -18.51658467707331113, 4.312655811444462195 ) ) ;
#6215=CARTESIAN_POINT ( 'NONE',  ( 199.0147604500337764, -12.44374936594963899, -15.65999889774876941 ) ) ;
#6244=CARTESIAN_POINT ( 'NONE',  ( 200.0000000000000000, 16.44874601624584187, 9.522804452304930223 ) ) ;
#6250=CARTESIAN_POINT ( 'NONE',  ( -192.9588430854689989, 10.23066800230756712, -10.23066800230735396 ) ) ;
#6251=CARTESIAN_POINT ( 'NONE',  ( 199.0210534451952924, 5.480999013853959489, 19.23967134089702569 ) ) ;
#6265=CARTESIAN_POINT ( 'NONE',  ( -213.1075012329537230, 9.698598906450543566, -9.698598906450348167 ) ) ;
#6275=CARTESIAN_POINT ( 'NONE',  ( 200.0000000000000000, 18.57749355353195497, -3.991677856843532712 ) ) ;
#6281=CARTESIAN_POINT ( 'NONE',  ( 199.0101504891794946, -4.065683697617192394, -19.58013257009994135 ) ) ;
#6288=CARTESIAN_POINT ( 'NONE',  ( 199.0216355752872914, 4.216131936211398035, 19.55614661669859444 ) ) ;
#6312=CARTESIAN_POINT ( 'NONE',  ( 200.0000000000000000, 18.87777001997802628, 2.191952217553565507 ) ) ;
#6313=CARTESIAN_POINT ( 'NONE',  ( 199.9999999999999432, -17.32226549516795089, -7.848194971284391031 ) ) ;
#6322=CARTESIAN_POINT ( 'NONE',  ( 199.0254345294016503, -6.947174024697130967, 18.76024293726333170 ) ) ;
#6323=CIRCLE ( 'NONE', #1660, 20.00000000000001421 ) ;
#6324=CARTESIAN_POINT ( 'NONE',  ( -56.48582580120559982, 50.09629031063956717, 6.472252184284792875 ) ) ;
#6326=CARTESIAN_POINT ( 'NONE',  ( 151.7948205124836534, 33.06932595376333239, 23.49921654116065284 ) ) ;
#6338=CARTESIAN_POINT ( 'NONE',  ( 199.0079861221352360, 1.294590733001960592, -19.95474696286750671 ) ) ;
#6367=CARTESIAN_POINT ( 'NONE',  ( 200.0000000000001137, 18.84395317400427317, -2.458366139920278304 ) ) ;
#6373=CARTESIAN_POINT ( 'NONE',  ( -192.9588430854690273, -18.05360324515400094, -38.51493924976961836 ) ) ;
#6374=CARTESIAN_POINT ( 'NONE',  ( 199.0261461916015264, -10.84957391917088110, 16.80813345823991867 ) ) ;
#6389=CARTESIAN_POINT ( 'NONE',  ( 199.0262408397048262, -11.66336112630027877, 16.25405011469380057 ) ) ;
#6402=CARTESIAN_POINT ( 'NONE',  ( 200.0000000000000000, -9.238661743929142744, 16.61727401759219092 ) ) ;
#6408=CARTESIAN_POINT ( 'NONE',  ( 199.0255278052971732, -18.60593281614774952, 7.356242102916651149 ) ) ;
#6420=CARTESIAN_POINT ( 'NONE',  ( 199.0053389886216451, 13.17958853561047228, -15.05032186847045672 ) ) ;
#6433=CARTESIAN_POINT ( 'NONE',  ( 199.0072917153253229, 3.369890617853546377, -19.72057389405671657 ) ) ;
#6445=CARTESIAN_POINT ( 'NONE',  ( 199.9999999999998863, -2.943496653232010374, -18.77345647985907462 ) ) ;
#6446=CARTESIAN_POINT ( 'NONE',  ( 200.0000000000000284, 12.52648961991985033, -14.29954643281654469 ) ) ;
#6456=CARTESIAN_POINT ( 'NONE',  ( 199.0118448083844385, 18.52953444905362090, 7.521846903409109331 ) ) ;
#6457=CARTESIAN_POINT ( 'NONE',  ( 192.4448373802100889, 14.14213562370330379, -14.14213562370292365 ) ) ;
#6459=CARTESIAN_POINT ( 'NONE',  ( -213.1075012329537230, 66.26714140138673770, -9.698598906462034819 ) ) ;
#6474=CARTESIAN_POINT ( 'NONE',  ( 199.0255278052971732, -18.60593281614774952, 7.356242102916651149 ) ) ;
#6502=CARTESIAN_POINT ( 'NONE',  ( 199.9999999999999716, 15.97866926103663765, -10.28159943737610860 ) ) ;
#6508=CARTESIAN_POINT ( 'NONE',  ( 199.0257180514102799, -8.261434504147922908, 18.22213678534573589 ) ) ;
#6539=CARTESIAN_POINT ( 'NONE',  ( 199.0258841556672564, -17.79651494919816912, 9.142457329253240061 ) ) ;
#6550=CARTESIAN_POINT ( 'NONE',  ( 199.0056040927672711, 16.99126215759308778, -10.54120702991739122 ) ) ;
#6563=CARTESIAN_POINT ( 'NONE',  ( 199.0119122942934098, -7.649365998490048391, -18.47719605185541170 ) ) ;
#6575=CARTESIAN_POINT ( 'NONE',  ( 199.9999999999999716, -3.557237102606629620, -18.66704445460036865 ) ) ;
#6577=CARTESIAN_POINT ( 'NONE',  ( 200.0000000000000284, 4.312859453180151625, -18.51524271434543323 ) ) ;
#6586=CARTESIAN_POINT ( 'NONE',  ( -91.56559293963834989, -44.31723036834885932, -12.25131212657538171 ) ) ;
#6601=CARTESIAN_POINT ( 'NONE',  ( 199.0214947048457077, -19.49260886005912141, -4.535603965114707314 ) ) ;
#6634=CARTESIAN_POINT ( 'NONE',  ( 200.0000000000000284, 8.678546691382686973, -16.90316441639222944 ) ) ;
#6637=CARTESIAN_POINT ( 'NONE',  ( -56.48582580120559982, -34.75652343174584047, -21.81201906317815187 ) ) ;
#6638=CARTESIAN_POINT ( 'NONE',  ( 199.0112867096082141, 18.93484222638594616, 6.440921653838688421 ) ) ;
#6672=CARTESIAN_POINT ( 'NONE',  ( 199.0193324171001450, -17.94164708558885124, -8.847044913458905313 ) ) ;
#6683=CARTESIAN_POINT ( 'NONE',  ( 199.0127395736742244, 17.77917978336349236, 9.157720830221606434 ) ) ;
#6699=CARTESIAN_POINT ( 'NONE',  ( 199.0059792703121389, 8.401033297471425243, -18.14527037458064385 ) ) ;
#6709=CARTESIAN_POINT ( 'NONE',  ( 199.9999999999998010, 5.803429233430792422, -18.09525674440013177 ) ) ;
#6722=CARTESIAN_POINT ( 'NONE',  ( 199.0132120035298442, 17.35012746940816797, 9.967304425461927408 ) ) ;
#6723=CARTESIAN_POINT ( 'NONE',  ( -192.9588430854689989, 10.23066800230756712, -10.23066800230735396 ) ) ;
#6733=ORIENTED_EDGE ( 'NONE', *, *, #26161, .F. ) ;
#6739=CARTESIAN_POINT ( 'NONE',  ( 199.0205186365099905, -18.88915341724846542, -6.581556047429298673 ) ) ;
#6767=CARTESIAN_POINT ( 'NONE',  ( 199.9999999999998010, 6.097523047862603462, -17.99825575681430223 ) ) ;
#6771=CARTESIAN_POINT ( 'NONE',  ( 19.06497207195980792, 10.03556273973447155, -10.03556273973422286 ) ) ;
#6772=CARTESIAN_POINT ( 'NONE',  ( 199.0103760074104002, 19.48024492545154018, 4.564568505664855280 ) ) ;
#6799=CARTESIAN_POINT ( 'NONE',  ( 199.9999999999999432, -8.412025548490841942, 17.05051154412392123 ) ) ;
#6804=CARTESIAN_POINT ( 'NONE',  ( 199.0176767632675023, -16.26464645690579758, -11.64139296301337190 ) ) ;
#6816=CARTESIAN_POINT ( 'NONE',  ( 199.0057363775755448, 17.49143510765091492, -9.692886659233986180 ) ) ;
#6830=CARTESIAN_POINT ( 'NONE',  ( 199.0063920675446525, 6.513768699308227106, -18.94368432171033945 ) ) ;
#6841=CARTESIAN_POINT ( 'NONE',  ( 199.9999999999998863, 9.229831349313808886, -16.61069465220444386 ) ) ;
#6843=CARTESIAN_POINT ( 'NONE',  ( 199.9999999999999147, 8.398447161810446815, -17.04410699012685271 ) ) ;
#6853=CARTESIAN_POINT ( 'NONE',  ( 199.0055953282818564, 16.96762334911333880, -10.59856222037965345 ) ) ;
#6854=CARTESIAN_POINT ( 'NONE',  ( 4.995406935893289102, 10.78321810389013002, -10.78321810388986712 ) ) ;
#6871=CARTESIAN_POINT ( 'NONE',  ( 199.0235864634049108, -19.99353228191618825, 0.6599136639449380004 ) ) ;
#6886=PLANE ( 'NONE',  #25922 ) ;
#6898=CARTESIAN_POINT ( 'NONE',  ( 200.0000000000001705, 6.971423609723053971, -17.67803530771774589 ) ) ;
#6902=CARTESIAN_POINT ( 'NONE',  ( 199.0183491629479988, 10.55513269831597079, 16.99244513920028510 ) ) ;
#6917=CARTESIAN_POINT ( 'NONE',  ( 19.06497207195980792, 10.03556273973447155, -10.03556273973422286 ) ) ;
#6919=ORIENTED_EDGE ( 'NONE', *, *, #15646, .T. ) ;
#6928=CARTESIAN_POINT ( 'NONE',  ( 199.9999999999999432, -5.384370329785186371, 18.23197071264586810 ) ) ;
#6933=CARTESIAN_POINT ( 'NONE',  ( 199.0228518427889242, -19.96294788386713037, -1.312843269464072815 ) ) ;
#6944=CARTESIAN_POINT ( 'NONE',  ( 199.0055466334479206, 16.72508833076945223, -10.95857635003404873 ) ) ;
#6960=CARTESIAN_POINT ( 'NONE',  ( 199.0110600102923115, -5.983788757275610770, -19.08445727264177094 ) ) ;
#6973=CARTESIAN_POINT ( 'NONE',  ( 199.9999999999998295, 1.074487055219422560, -18.97158139261448540 ) ) ;
#6983=CARTESIAN_POINT ( 'NONE',  ( 146.6084372240433709, -24.48358557860284179, -32.08495691632087699 ) ) ;
#6996=CARTESIAN_POINT ( 'NONE',  ( 199.0258841556672564, -17.79651494919816912, 9.142457329253240061 ) ) ;
#7024=CARTESIAN_POINT ( 'NONE',  ( 200.0000000000001990, 0.6082288760829889229, -18.99424756986708474 ) ) ;
#7028=CARTESIAN_POINT ( 'NONE',  ( 199.0181823811410311, 10.83083347386195427, 16.81793973133765618 ) ) ;
#7048=CARTESIAN_POINT ( 'NONE',  ( 199.0252416244725282, -6.134786337322394090, 19.04345623536530141 ) ) ;
#7050=CARTESIAN_POINT ( 'NONE',  ( 4.995406935893283773, 39.06748935135171052, 17.50105314357239195 ) ) ;
#7058=CARTESIAN_POINT ( 'NONE',  ( -105.3755690713226727, -15.38646221621807619, 15.38646221621768362 ) ) ;
#7068=CARTESIAN_POINT ( 'NONE',  ( 199.9999999999996589, -3.408648353384132079, 18.70401797595889448 ) ) ;
#7097=CARTESIAN_POINT ( 'NONE',  ( 199.0186487660832029, -17.30925014347549862, -10.04346281267784669 ) ) ;
#7107=CARTESIAN_POINT ( 'NONE',  ( 199.9999999999999432, -9.907006709245502307, -16.21817530592209522 ) ) ;
#7118=CARTESIAN_POINT ( 'NONE',  ( 184.8905102610680444, -14.79361573936330565, -41.77492675556016621 ) ) ;
#7131=CARTESIAN_POINT ( 'NONE',  ( 200.0000000000000568, 7.542793502284206753, 17.44923311141863920 ) ) ;
#7154=CARTESIAN_POINT ( 'NONE',  ( 199.9999999999999147, -3.403913688674531812, -18.69557029314349705 ) ) ;
#7158=CARTESIAN_POINT ( 'NONE',  ( 199.0189287881835583, 9.564175521352543896, 17.56735958655279362 ) ) ;
#7171=CARTESIAN_POINT ( 'NONE',  ( -86.96347745069644475, -15.38646221621807442, 15.38646221621768184 ) ) ;
#7187=CARTESIAN_POINT ( 'NONE',  ( 199.9999999999999716, -11.58333327279321701, 15.07704058621049548 ) ) ;
#7196=DIRECTION ( 'NONE',  ( -1.000000000000000000, -1.836970198721030181E-16, -2.465190328815661892E-32 ) ) ;
#7218=CARTESIAN_POINT ( 'NONE',  ( 199.0252574105521717, -19.02124966810586315, 6.202843364552198757 ) ) ;
#7229=CARTESIAN_POINT ( 'NONE',  ( 199.9999999999999716, -18.76480772196043034, -3.095184993347289026 ) ) ;
#7254=CARTESIAN_POINT ( 'NONE',  ( 199.9999999999996305, -4.934527571401590151, 18.35877764772902410 ) ) ;
#7280=CARTESIAN_POINT ( 'NONE',  ( 200.0000000000001990, -15.45587892757197146, -11.06220582312848144 ) ) ;
#7284=CARTESIAN_POINT ( 'NONE',  ( 199.0053389886216451, 13.17958853561047228, -15.05032186847045672 ) ) ;
#7306=ORIENTED_EDGE ( 'NONE', *, *, #11113, .T. ) ;
#7312=CARTESIAN_POINT ( 'NONE',  ( 199.9999999999999716, 1.225499021177249404, 18.97167928969624384 ) ) ;
#7343=CARTESIAN_POINT ( 'NONE',  ( 199.0199639038170574, -18.47329534536968509, -7.669176827176202416 ) ) ;
#7350=CARTESIAN_POINT ( 'NONE',  ( 170.2234770963711128, 10.92277846919216522, -10.92277846919186501 ) ) ;
#7352=CARTESIAN_POINT ( 'NONE',  ( 199.9999999999999147, -17.67734251759716457, -6.986728219496066927 ) ) ;
#7366=CARTESIAN_POINT ( 'NONE',  ( 136.1360204305621266, -24.77266263493151044, 24.77266263493093135 ) ) ;
#7379=CARTESIAN_POINT ( 'NONE',  ( 200.0000000000000000, 2.625635831523228880, 18.82681798050185051 ) ) ;
#7403=CARTESIAN_POINT ( 'NONE',  ( 200.0000000000001421, -10.69674284809226350, -15.70882504007707681 ) ) ;
#7405=CARTESIAN_POINT ( 'NONE',  ( 199.0055119247266759, 16.54204028020789252, -11.23294693469441263 ) ) ;
#7425=CARTESIAN_POINT ( 'NONE',  ( -56.48582580120559271, -6.472252184284276844, 6.472252184284108978 ) ) ;
#7436=CARTESIAN_POINT ( 'NONE',  ( 200.0000000000002842, -5.234650960127995134, 18.27551028936266775 ) ) ;
#7468=CARTESIAN_POINT ( 'NONE',  ( 199.0156711280681350, -13.74982657632009264, -14.52405353129264043 ) ) ;
#7479=CARTESIAN_POINT ( 'NONE',  ( 199.9999999999998579, -10.30558286630674658, -15.96802547070553047 ) ) ;
#7509=CARTESIAN_POINT ( 'NONE',  ( 200.0000000000000284, 9.630262036685882876, 16.38694142346205140 ) ) ;
#7525=CARTESIAN_POINT ( 'NONE',  ( 170.2234770963711128, -17.36149277827010096, 17.36149277826970660 ) ) ;
#7534=CARTESIAN_POINT ( 'NONE',  ( 199.9999999999998579, -16.14759498898286338, -10.02975912355057453 ) ) ;
#7537=CARTESIAN_POINT ( 'NONE',  ( 199.0054122081438948, 15.86953797770180508, -12.16778084942700211 ) ) ;
#7565=CARTESIAN_POINT ( 'NONE',  ( 199.9999999999995453, -10.04557064260861843, 16.14007440661455206 ) ) ;
#7597=CARTESIAN_POINT ( 'NONE',  ( 199.0224076953712711, -19.86590228279781201, -2.420100283956707621 ) ) ;
#7605=CARTESIAN_POINT ( 'NONE',  ( -56.48582580120559271, 21.81201906317798489, -21.81201906317746619 ) ) ;
#7607=CARTESIAN_POINT ( 'NONE',  ( 199.9999999999998863, -18.14641137086378819, -5.658975142792487922 ) ) ;
#7633=CARTESIAN_POINT ( 'NONE',  ( 199.9999999999998863, -4.328516665792998097, 18.51095020188552809 ) ) ;
#7634=CARTESIAN_POINT ( 'NONE',  ( 199.9999999999999716, -14.30114536083090471, 12.54040393066167347 ) ) ;
#7646=CARTESIAN_POINT ( 'NONE',  ( -162.0762913951021176, 57.76657433523994456, -1.198031840315424867 ) ) ;
#7649=CARTESIAN_POINT ( 'NONE',  ( -100.7734535825088358, -16.03295912088728770, 16.03295912088687913 ) ) ;
#7662=CARTESIAN_POINT ( 'NONE',  ( 200.0000000000001421, -14.29287298608315382, 12.53529920294169386 ) ) ;
#7665=CARTESIAN_POINT ( 'NONE',  ( 199.0062089136474128, 7.336486126005011599, -18.60345363517511430 ) ) ;
#7684=CARTESIAN_POINT ( 'NONE',  ( 130.8568914410475372, -24.07718906447255947, 24.07718906447199458 ) ) ;
#7696=CARTESIAN_POINT ( 'NONE',  ( 199.9999999999999716, 17.67160698027466736, 6.995183481556395577 ) ) ;
#7703=CARTESIAN_POINT ( 'NONE',  ( 0.2972598230770011618, 10.13633138497555919, -66.70487387989845729 ) ) ;
#7739=CARTESIAN_POINT ( 'NONE',  ( 199.0241407150285227, -2.291925048877014870, 19.87495682421008425 ) ) ;
#7767=CARTESIAN_POINT ( 'NONE',  ( 199.9999999999996874, 13.64679526057751069, 13.22824625860694070 ) ) ;
#7768=CARTESIAN_POINT ( 'NONE',  ( 200.0000000000000284, -18.10041568647748278, 5.811528243237751745 ) ) ;
#7778=CARTESIAN_POINT ( 'NONE',  ( 199.0155675229561609, 14.66025079576549750, 13.60702933000608006 ) ) ;
#7779=CARTESIAN_POINT ( 'NONE',  ( -238.4067589809705794, 57.25054294065799354, -0.6820004457334954973 ) ) ;
#7782=CARTESIAN_POINT ( 'NONE',  ( -213.1075012329537230, 37.98287015391211696, 18.58567234101190735 ) ) ;
#7791=CARTESIAN_POINT ( 'NONE',  ( 199.9999999999996874, -18.85616045826023779, 2.487226269395955480 ) ) ;
#7795=CARTESIAN_POINT ( 'NONE',  ( 199.0112868605082497, -6.441215115722609852, -18.93473387006624620 ) ) ;
#7822=ORIENTED_EDGE ( 'NONE', *, *, #17819, .F. ) ;
#7823=CARTESIAN_POINT ( 'NONE',  ( 199.9999999999999432, 18.93973332185608172, 1.567235916626209535 ) ) ;
#7831=CARTESIAN_POINT ( 'NONE',  ( -91.56559293963834989, 12.25131212657497848, -12.25131212657469426 ) ) ;
#7861=CARTESIAN_POINT ( 'NONE',  ( 199.9999999999999716, 18.66316687947711728, 3.577466338041057181 ) ) ;
#7867=CARTESIAN_POINT ( 'NONE',  ( 199.0072281836893637, 3.578240568248503894, -19.67355276342582115 ) ) ;
#7872=CARTESIAN_POINT ( 'NONE',  ( 200.0000000000001421, -14.29287298608315382, 12.53529920294169386 ) ) ;
#7877=CARTESIAN_POINT ( 'NONE',  ( 199.0137418305357073, 16.79925839223816197, 10.85573510210755899 ) ) ;
#7905=CARTESIAN_POINT ( 'NONE',  ( 200.0000000000000853, 18.51119012207909620, 4.337730402235636440 ) ) ;
#7906=CARTESIAN_POINT ( 'NONE',  ( 199.9999999999999147, -15.18276431615445610, 11.44766049767000915 ) ) ;
#7917=CARTESIAN_POINT ( 'NONE',  ( 199.0224155992051180, 2.400915676194647741, 19.86821540553048848 ) ) ;
#7918=CARTESIAN_POINT ( 'NONE',  ( -56.48582580120559982, -6.472252184283581400, -50.09629031063973059 ) ) ;
#7933=CARTESIAN_POINT ( 'NONE',  ( 200.0000000000001421, -15.08701489606589341, 11.56722645162647467 ) ) ;
#7936=CARTESIAN_POINT ( 'NONE',  ( 199.0117582043400830, -7.359043231587310885, -18.59750019459799120 ) ) ;
#7963=CARTESIAN_POINT ( 'NONE',  ( 199.9999999999999147, 6.094537134382843391, 18.00666549647224812 ) ) ;
#7969=CARTESIAN_POINT ( 'NONE',  ( -162.0762913951020892, 29.48230308784799902, -29.48230308784730980 ) ) ;
#7970=CARTESIAN_POINT ( 'NONE',  ( 199.0228608363770206, 1.289830063590766907, 19.96444201077071057 ) ) ;
#7971=APPLICATION_CONTEXT ( 'automotive_design' ) ;
#7994=CARTESIAN_POINT ( 'NONE',  ( 0.000000000000000000, 0.000000000000000000, 0.000000000000000000 ) ) ;
#7997=CARTESIAN_POINT ( 'NONE',  ( 199.9999999999999432, 17.99246019556983711, 6.122134764576554034 ) ) ;
#8004=CARTESIAN_POINT ( 'NONE',  ( 199.0095093599360894, -2.612260778589423182, -19.82812366214328748 ) ) ;
#8015=CARTESIAN_POINT ( 'NONE',  ( 199.0248237628271113, -4.554872532684343334, 19.47958378538321611 ) ) ;
#8042=CARTESIAN_POINT ( 'NONE',  ( 200.0000000000000568, 16.12943746570313053, 10.05448153537135347 ) ) ;
#8044=CARTESIAN_POINT ( 'NONE',  ( 199.9999999999999432, -15.98279859272680170, -10.29025366354621696 ) ) ;
#8055=CARTESIAN_POINT ( 'NONE',  ( -91.56559293963834989, 12.25131212657497848, -12.25131212657469426 ) ) ;
#8057=CARTESIAN_POINT ( 'NONE',  ( -30.26275506840324070, 1.198031551616030033, -1.198031551616006496 ) ) ;
#8066=CARTESIAN_POINT ( 'NONE',  ( 199.9999999999999716, -17.78976893299991247, -6.695511796223322598 ) ) ;
#8070=CARTESIAN_POINT ( 'NONE',  ( 199.0106728332879698, -5.188592077825961546, -19.31531804097554073 ) ) ;
#8099=CARTESIAN_POINT ( 'NONE',  ( 199.9999999999999432, 14.48708306876533136, 12.30466461812483914 ) ) ;
#8105=CARTESIAN_POINT ( 'NONE',  ( 19.06497207195981858, 10.03556273973516078, -66.60410523465806421 ) ) ;
#8106=CARTESIAN_POINT ( 'NONE',  ( 199.0259813356335883, -9.719824439858887999, 17.48565896982476175 ) ) ;
#8136=CARTESIAN_POINT ( 'NONE',  ( 199.9999999999999716, 18.87797660738322847, 2.189960623836138875 ) ) ;
#8142=CARTESIAN_POINT ( 'NONE',  ( 199.0061077845142279, 7.790749371913985755, -18.41559517569303495 ) ) ;
#8148=CARTESIAN_POINT ( 'NONE',  ( 200.0000000000005400, -16.47398309245309278, 9.506867245997410620 ) ) ;
#8152=CARTESIAN_POINT ( 'NONE',  ( 199.0224671581742371, 2.272106995489924230, 19.87442369886018767 ) ) ;
#8179=CARTESIAN_POINT ( 'NONE',  ( 199.9999999999999716, 15.96353534131429797, 10.31599105002992545 ) ) ;
#8180=CARTESIAN_POINT ( 'NONE',  ( 199.9999999999999147, -11.07985673941785976, -15.44349624739909643 ) ) ;
#8190=CARTESIAN_POINT ( 'NONE',  ( 199.0199803820819966, 7.637620434976441608, 18.48637365640330188 ) ) ;
#8191=CARTESIAN_POINT ( 'NONE',  ( -198.0356074513804572, 39.15871834505956173, -39.15871834505865223 ) ) ;
#8193=CARTESIAN_POINT ( 'NONE',  ( 57.59792236341147031, 54.84617931850878136, 1.722363176415705910 ) ) ;
#8196=EDGE_LOOP ( 'NONE', ( #24874, #16484 ) ) ;
#8201=CARTESIAN_POINT ( 'NONE',  ( 199.9999999999996589, -18.76526504493254777, 3.099636891498418478 ) ) ;
#8204=CARTESIAN_POINT ( 'NONE',  ( 199.0078145870362221, 1.786107411569149317, -19.91668635079984284 ) ) ;
#8231=CARTESIAN_POINT ( 'NONE',  ( 199.9999999999998863, 8.393744152662998559, 17.05383455604227905 ) ) ;
#8237=CARTESIAN_POINT ( 'NONE',  ( -86.96347745069644475, 12.89780903124419353, -12.89780903124389333 ) ) ;
#8238=CARTESIAN_POINT ( 'NONE',  ( 199.0262910934941942, -12.18938195246538037, 15.86593956234834479 ) ) ;
#8263=CARTESIAN_POINT ( 'NONE',  ( 200.0000000000000000, 8.256023932303243384, 17.12527061769673153 ) ) ;
#8270=CARTESIAN_POINT ( 'NONE',  ( 199.0060114145493912, 8.242208747961328186, -18.21796198456784666 ) ) ;
#8278=CARTESIAN_POINT ( 'NONE',  ( 199.0176798082135008, 11.64390658120213828, 16.27508030683247497 ) ) ;
#8298=CIRCLE ( 'NONE', #14656, 10.00000000000000000 ) ;
#8305=CARTESIAN_POINT ( 'NONE',  ( 199.9999999999998579, 13.31531350134012648, 13.56203446005050317 ) ) ;
#8307=CARTESIAN_POINT ( 'NONE',  ( 199.9999999999999716, -18.96854328187948369, -1.244406218240217799 ) ) ;
#8319=CARTESIAN_POINT ( 'NONE',  ( 130.8568914410475088, 32.49135343045448820, 24.07718906446946860 ) ) ;
#8321=CARTESIAN_POINT ( 'NONE',  ( -198.0356074513804572, 67.44298959250878056, -10.87444709758402261 ) ) ;
#8331=ORIENTED_EDGE ( 'NONE', *, *, #25405, .F. ) ;
#8338=CARTESIAN_POINT ( 'NONE',  ( 199.0166470710653925, -15.03895783737594805, -13.18902814565699266 ) ) ;
#8365=CARTESIAN_POINT ( 'NONE',  ( 200.0000000000001421, 16.91347576093571803, -8.662591770200990027 ) ) ;
#8372=CARTESIAN_POINT ( 'NONE',  ( -208.1127848780264742, -17.67593391476605547, -38.89260858015755673 ) ) ;
#8373=CARTESIAN_POINT ( 'NONE',  ( 199.0259577874143417, -9.576177499050416486, 17.56472219104047028 ) ) ;
#8386=CARTESIAN_POINT ( 'NONE',  ( -162.0762913951020892, 1.198031840385732849, -1.198031840385733515 ) ) ;
#8396=CARTESIAN_POINT ( 'NONE',  ( 199.9999999999998863, 17.79007744789355172, -6.680419707818059827 ) ) ;
#8402=CARTESIAN_POINT ( 'NONE',  ( 199.0142478014330720, -11.65985798941387941, -16.24932773989132073 ) ) ;
#8406=EDGE_CURVE ( 'NONE', #5454, #122, #26156, .T. ) ;
#8413=CARTESIAN_POINT ( 'NONE',  ( 199.0095182511445557, 19.82538855659994681, 2.633105091475395287 ) ) ;
#8420=DIRECTION ( 'NONE',  ( 0.000000000000000000, -1.000000000000000000, 0.000000000000000000 ) ) ;
#8441=CARTESIAN_POINT ( 'NONE',  ( 200.0000000000000568, 2.475862818518347552, -18.83975305017670365 ) ) ;
#8442=CARTESIAN_POINT ( 'NONE',  ( 199.9999999999999147, -1.249805991376689018, -18.96320409372175675 ) ) ;
#8453=CARTESIAN_POINT ( 'NONE',  ( 136.1360204305621266, 3.511608612530757068, -3.511608612530642937 ) ) ;
#8455=CARTESIAN_POINT ( 'NONE',  ( -105.3755690713226585, 12.89780903124349720, 43.67073346367994446 ) ) ;
#8468=CARTESIAN_POINT ( 'NONE',  ( 199.0257179982615128, -18.22226585379655361, 8.261159732268383848 ) ) ;
#8494=AXIS2_PLACEMENT_3D ( 'NONE', #2297, #22402, #15992 ) ;
#8501=CARTESIAN_POINT ( 'NONE',  ( 200.0000000000002842, 18.39723030902092660, -4.753359243483134655 ) ) ;
#8506=CARTESIAN_POINT ( 'NONE',  ( 14.38125909742180752, 10.73282306404735387, -10.73282306404708919 ) ) ;
#8519=CARTESIAN_POINT ( 'NONE',  ( 199.0261637166634330, -10.98746419350304748, 16.71832627740758070 ) ) ;
#8539=CARTESIAN_POINT ( 'NONE',  ( 199.0214947048457077, -19.49260886005912141, -4.535603965114707314 ) ) ;
#8551=CARTESIAN_POINT ( 'NONE',  ( 199.0085879884812243, 19.99611484057871280, 0.3390174452003563710 ) ) ;
#8566=CARTESIAN_POINT ( 'NONE',  ( 199.0060256982278588, 8.174003731485944613, -18.24926009350555134 ) ) ;
#8576=B_SPLINE_CURVE_WITH_KNOTS ( 'NONE', 3,
 ( #9472, #25852, #15708, #23833, #5615, #13721, #24380, #9870, #10136, #12391, #26261, #8396, #1898, #5744, #16252, #10003, #17973, #6275, #18380, #5881, #1762, #3899, #16115, #26119, #2288, #23968, #25, #13849, #18240, #8136, #21984, #24245, #18110, #7861, #3755, #22120, #6018, #7997, #15980, #20253, #14126, #20516, #289, #6144, #4169, #11997, #22254, #4031, #14255, #24108, #10396, #22393, #12263, #12131, #13988, #20120, #2034, #20387, #11860, #18511, #19980, #2162, #10272, #159, #8263, #16383, #24516, #14390, #22521, #4301, #2698, #25048, #4424, #14643, #12929, #24914, #695, #16913, #8801, #15045, #18781, #12657, #21178, #25178, #564, #12517, #10803, #10937, #14518, #6928, #2422, #17043, #8668, #22782, #6799, #20783, #6402, #23176, #18913, #4955, #10531, #2554, #2952, #14910, #4561, #18644, #23052, #10670 ),
 .UNSPECIFIED., .F., .F.,
 ( 4, 2, 1, 2, 2, 2, 2, 2, 1, 2, 2, 2, 2, 2, 2, 2, 1, 2, 2, 2, 2, 2, 1, 2, 2, 2, 2, 2, 2, 2, 2, 2, 2, 2, 1, 2, 2, 2, 1, 2, 2, 2, 2, 2, 2, 2, 1, 2, 2, 2, 2, 2, 1, 2, 2, 2, 2, 4 ),
 ( 0.5000000000000000000, 0.5312500000000004441, 0.5390625000000005551, 0.5429687500000005551, 0.5468750000000005551, 0.5625000000000005551, 0.5703125000000005551, 0.5781250000000005551, 0.5859375000000005551, 0.5898437500000006661, 0.5937500000000006661, 0.6015625000000006661, 0.6093750000000006661, 0.6171875000000007772, 0.6250000000000007772, 0.6406250000000008882, 0.6484375000000008882, 0.6523437500000008882, 0.6562500000000008882, 0.6718750000000008882, 0.6796875000000008882, 0.6875000000000008882, 0.6953125000000008882, 0.6992187500000008882, 0.7031250000000009992, 0.7187500000000008882, 0.7265625000000008882, 0.7343750000000008882, 0.7500000000000008882, 0.7578125000000008882, 0.7656250000000008882, 0.7812500000000008882, 0.7890625000000008882, 0.7968750000000008882, 0.8046875000000008882, 0.8085937500000008882, 0.8125000000000008882, 0.8281250000000008882, 0.8359375000000008882, 0.8398437500000007772, 0.8437500000000006661, 0.8515625000000006661, 0.8593750000000006661, 0.8671875000000005551, 0.8750000000000004441, 0.9062500000000002220, 0.9140625000000002220, 0.9179687500000001110, 0.9218750000000000000, 0.9375000000000000000, 0.9453125000000000000, 0.9531250000000000000, 0.9609375000000000000, 0.9648437500000000000, 0.9687500000000000000, 0.9765625000000000000, 0.9843750000000000000, 1.000000000000000000 ),
 .UNSPECIFIED. ) ;
#8579=CARTESIAN_POINT ( 'NONE',  ( 199.9999999999999716, 15.97866926103663765, -10.28159943737610860 ) ) ;
#8592=CARTESIAN_POINT ( 'NONE',  ( 91.82158438592158234, -40.45024623143936537, -16.11829626348475131 ) ) ;
#8594=CARTESIAN_POINT ( 'NONE',  ( -30.26275506840325136, 29.48230279907760121, 27.08623969584625613 ) ) ;
#8608=CARTESIAN_POINT ( 'NONE',  ( 199.9999999999999716, -11.58333327279321701, 15.07704058621049548 ) ) ;
#8635=CARTESIAN_POINT ( 'NONE',  ( 199.9999999999998295, 8.257913856993376100, -17.11264870637372226 ) ) ;
#8639=CARTESIAN_POINT ( 'NONE',  ( -105.3755690713226585, -43.67073346367964604, -12.89780903124457545 ) ) ;
#8640=CARTESIAN_POINT ( 'NONE',  ( 199.0164010208656009, 13.53619804287660777, 14.72436343555392035 ) ) ;
#8668=CARTESIAN_POINT ( 'NONE',  ( 199.9999999999999432, -7.568351747471193214, 17.44130164783803139 ) ) ;
#8675=CARTESIAN_POINT ( 'NONE',  ( 199.0238156666156044, -19.96322609118500324, 1.315852278599464631 ) ) ;
#8688=CARTESIAN_POINT ( 'NONE',  ( 199.0060120359516986, 18.22327268582330007, -8.235267977567980680 ) ) ;
#8702=CARTESIAN_POINT ( 'NONE',  ( -265.0000000000000000, 9.999999999999952038, 1.224646799147346551E-15 ) ) ;
#8711=CARTESIAN_POINT ( 'NONE',  ( -265.0000000000000000, 9.999999999999952038, 1.224646799147346551E-15 ) ) ;
#8712=CARTESIAN_POINT ( 'NONE',  ( 199.9999999999998863, 12.52392839731578889, -14.30162278802013098 ) ) ;
#8713=CARTESIAN_POINT ( 'NONE',  ( 199.9999999999999147, 3.090567748620505650, -18.74862269653256419 ) ) ;
#8722=CARTESIAN_POINT ( 'NONE',  ( 199.0078462942310296, 19.92684364972848243, -1.695029663804312303 ) ) ;
#8723=CARTESIAN_POINT ( 'NONE',  ( 19.06497207195980792, -18.24870850772710540, -38.31983398719647482 ) ) ;
#8739=CARTESIAN_POINT ( 'NONE',  ( 199.0242480509055270, -19.84286657041863933, 2.617213520271152394 ) ) ;
#8765=VERTEX_POINT ( 'NONE', #5623 ) ;
#8768=CARTESIAN_POINT ( 'NONE',  ( 200.0000000000000000, 15.45062812681867825, -11.05917137904152625 ) ) ;
#8772=CARTESIAN_POINT ( 'NONE',  ( -259.2033419157646676, -6.730120644403663199, 6.730120644403451813 ) ) ;
#8773=CARTESIAN_POINT ( 'NONE',  ( 199.0157948715101668, 14.36126147255820484, 13.92041998760680066 ) ) ;
#8801=CARTESIAN_POINT ( 'NONE',  ( 199.9999999999999147, 2.157212532375118563, 18.88823879575998177 ) ) ;
#8807=CARTESIAN_POINT ( 'NONE',  ( 199.0191706476670959, -17.79509468669765226, -9.138050845474172235 ) ) ;
#8819=CARTESIAN_POINT ( 'NONE',  ( 199.0067627483201989, 19.31843298438769807, -5.161535144790875940 ) ) ;
#8836=CARTESIAN_POINT ( 'NONE',  ( 199.0061118454574114, 7.773422122678746327, -18.42227132588763183 ) ) ;
#8847=CARTESIAN_POINT ( 'NONE',  ( 199.9999999999999716, 7.832101404672591194, -17.31171755797958056 ) ) ;
#8848=CARTESIAN_POINT ( 'NONE',  ( 199.9999999999999147, -9.095991256943364078, -16.68624471194709358 ) ) ;
#8856=CARTESIAN_POINT ( 'NONE',  ( 199.0061137528103359, 18.42594117564502909, -7.764722426784522291 ) ) ;
#8857=CARTESIAN_POINT ( 'NONE',  ( 0.2972598230769990524, -18.14793986248671231, -38.42060263243687501 ) ) ;
#8873=CARTESIAN_POINT ( 'NONE',  ( 199.0263771350486763, -14.37646237564524476, 13.91501816527019919 ) ) ;
#8899=CARTESIAN_POINT ( 'NONE',  ( 199.9999999999996021, 9.500464834803043601, -16.45734938164063621 ) ) ;
#8903=CARTESIAN_POINT ( 'NONE',  ( -100.7734535825088500, -44.31723036834885932, -12.25131212657538171 ) ) ;
#8904=CARTESIAN_POINT ( 'NONE',  ( 199.0111318983613842, 19.03723981379789265, 6.131360352008743853 ) ) ;
#8921=CARTESIAN_POINT ( 'NONE',  ( 170.2234770963711128, 10.92277846919147066, 45.64576402573197811 ) ) ;
#8942=CARTESIAN_POINT ( 'NONE',  ( 199.0170773700648397, -15.56690153483635264, -12.55869779031424116 ) ) ;
#8954=CARTESIAN_POINT ( 'NONE',  ( 199.0053905349878107, 15.66748078252780374, -12.42684713134076979 ) ) ;
#8969=CARTESIAN_POINT ( 'NONE',  ( 199.0094080386897986, -2.402341955940460405, -19.89500313782861696 ) ) ;
#8980=CARTESIAN_POINT ( 'NONE',  ( 200.0000000000000853, 3.093441846007485285, -18.74813587279223981 ) ) ;
#8982=CARTESIAN_POINT ( 'NONE',  ( 199.9999999999999147, 7.976971673177774669, -17.24969891087616602 ) ) ;
#8993=CARTESIAN_POINT ( 'NONE',  ( 199.0118837125828861, 18.49943804575643824, 7.595438918186243171 ) ) ;
#8994=CARTESIAN_POINT ( 'NONE',  ( 91.82158438592158234, -12.16597498397778843, 12.16597498397750954 ) ) ;
#9008=CARTESIAN_POINT ( 'NONE',  ( 199.0212029771548430, -19.33411866963394488, -5.169619751639646488 ) ) ;
#9035=CARTESIAN_POINT ( 'NONE',  ( 199.9999999999999147, -10.82539530975288855, -15.62049148088690131 ) ) ;
#9039=CARTESIAN_POINT ( 'NONE',  ( 199.0122446118616892, 18.20979473430505280, 8.267810710173087330 ) ) ;
#9052=CARTESIAN_POINT ( 'NONE',  ( 199.0259577874143417, -9.576177499050416486, 17.56472219104047028 ) ) ;
#9054=CARTESIAN_POINT ( 'NONE',  ( 192.4448373802101173, 14.14213562370261279, 42.42640687122091236 ) ) ;
#9068=CARTESIAN_POINT ( 'NONE',  ( 199.0235864634049108, -19.99353228191618825, 0.6599136639449380004 ) ) ;
#9095=CARTESIAN_POINT ( 'NONE',  ( 199.0231574205945435, -19.99787883075954653, -0.5143984472968653465 ) ) ;
#9103=CARTESIAN_POINT ( 'NONE',  ( 199.9999999999996305, -13.87326568555608830, -12.99368172854615366 ) ) ;
#9113=CARTESIAN_POINT ( 'NONE',  ( -198.0356074513804572, -17.40982414986427429, -39.15871834505933435 ) ) ;
#9126=CARTESIAN_POINT ( 'NONE',  ( 199.9999999999998579, 2.934899133129863280, 18.78102297366244500 ) ) ;
#9157=CARTESIAN_POINT ( 'NONE',  ( 199.9999999999999432, -6.993216068016765874, -17.67234381275832433 ) ) ;
#9160=CARTESIAN_POINT ( 'NONE',  ( 199.0079837170424923, 19.96494570524563272, -1.290871210190707608 ) ) ;
#9178=CARTESIAN_POINT ( 'NONE',  ( -162.0762913951021176, 29.48230308784730980, 27.08623940707652622 ) ) ;
#9184=CARTESIAN_POINT ( 'NONE',  ( 19.06497207195980792, 10.03556273973447155, -10.03556273973422286 ) ) ;
#9193=CARTESIAN_POINT ( 'NONE',  ( 200.0000000000000000, -12.54535540268124372, 14.29661512548269187 ) ) ;
#9224=CARTESIAN_POINT ( 'NONE',  ( 199.0254832151936171, -18.68063995892892137, 7.159751105900188151 ) ) ;
#9236=CARTESIAN_POINT ( 'NONE',  ( 199.9999999999999716, -6.704437273156823807, -17.78382994799445527 ) ) ;
#9261=CARTESIAN_POINT ( 'NONE',  ( 199.9999999999996589, 6.678198862535981384, 17.79829383751451388 ) ) ;
#9284=CARTESIAN_POINT ( 'NONE',  ( 200.0000000000002558, 2.008769787671115026, -18.89534854373681938 ) ) ;
#9290=CARTESIAN_POINT ( 'NONE',  ( 199.0060114145493912, 8.242208747961328186, -18.21796198456784666 ) ) ;
#9318=CARTESIAN_POINT ( 'NONE',  ( 199.9999999999998295, 0.2943743412949595961, 19.00910698902408669 ) ) ;
#9348=CARTESIAN_POINT ( 'NONE',  ( 199.0196838869227633, -18.24539314265820877, -8.197241283090187736 ) ) ;
#9355=CARTESIAN_POINT ( 'NONE',  ( 151.7948205124836250, 4.785054706301759886, -4.785054706301612448 ) ) ;
#9357=CARTESIAN_POINT ( 'NONE',  ( 200.0000000000000000, -19.00702131438069031, 0.3144861700050793352 ) ) ;
#9384=CARTESIAN_POINT ( 'NONE',  ( 200.0000000000001421, 9.088304224312857116, 16.69380151103622012 ) ) ;
#9412=CARTESIAN_POINT ( 'NONE',  ( 199.9999999999999716, -15.72304121538119936, -10.67928908684366540 ) ) ;
#9415=CARTESIAN_POINT ( 'NONE',  ( 199.0055623607443636, 10.83365079593514757, -16.80863377785637169 ) ) ;
#9433=CARTESIAN_POINT ( 'NONE',  ( -198.0356074513804572, 10.87444709759730088, -10.87444709759707173 ) ) ;
#9445=CARTESIAN_POINT ( 'NONE',  ( 199.9999999999999432, -7.567711247534615993, 17.44155761536767812 ) ) ;
#9472=CARTESIAN_POINT ( 'NONE',  ( 199.9999999999998863, 13.43021917686961331, -13.43983678748323918 ) ) ;
#9473=CARTESIAN_POINT ( 'NONE',  ( 199.0263771574038856, -15.03208543695887300, 13.25939591991213717 ) ) ;
#9483=CARTESIAN_POINT ( 'NONE',  ( -162.0762913951020892, 29.48230308784799902, -29.48230308784730980 ) ) ;
#9485=CARTESIAN_POINT ( 'NONE',  ( 200.0000000000001137, -18.99355687379454949, 0.7833857536329088544 ) ) ;
#9511=CARTESIAN_POINT ( 'NONE',  ( 199.9999999999998863, 6.967860089407453827, 17.68684069956508154 ) ) ;
#9524=CARTESIAN_POINT ( 'NONE',  ( -198.0356074513804572, 10.87444709759730088, -10.87444709759707173 ) ) ;
#9533=CARTESIAN_POINT ( 'NONE',  ( 199.9999999999999147, -14.49496992596536771, -12.29673964441684042 ) ) ;
#9537=CARTESIAN_POINT ( 'NONE',  ( 199.0054956575951621, 16.44889389956343706, -11.36889162147346255 ) ) ;
#9539=UNCERTAINTY_MEASURE_WITH_UNIT (LENGTH_MEASURE( 1.000000000000000082E-05 ), #1206, 'distance_accuracy_value', 'NONE');
#9568=CARTESIAN_POINT ( 'NONE',  ( 200.0000000000001990, -4.022463818607304731, 18.57981244883409744 ) ) ;
#9587=LINE ( 'NONE', #13573, #11699 ) ;
#9618=CARTESIAN_POINT ( 'NONE',  ( 199.9999999999999147, -10.43683117453143261, -15.88259547814976180 ) ) ;
#9646=CARTESIAN_POINT ( 'NONE',  ( 199.9999999999999147, 0.6045081272180472531, 19.00173049909658474 ) ) ;
#9647=CARTESIAN_POINT ( 'NONE',  ( 200.0000000000000000, -13.88319085540579678, 13.00159729487775451 ) ) ;
#9659=CARTESIAN_POINT ( 'NONE',  ( 163.1118516004056573, 9.006482792073693844, 47.56205970284970164 ) ) ;
#9671=CARTESIAN_POINT ( 'NONE',  ( 200.0000000000000284, -14.89458464808834748, 11.81399803044240038 ) ) ;
#9674=CARTESIAN_POINT ( 'NONE',  ( 199.0059208051008852, 8.690306674284110855, -18.00847358856242408 ) ) ;
#9691=CARTESIAN_POINT ( 'NONE',  ( 91.82158438592158234, -12.16597498397778843, 12.16597498397750954 ) ) ;
#9702=CARTESIAN_POINT ( 'NONE',  ( 199.9999999999998863, -4.328516665792998097, 18.51095020188552809 ) ) ;
#9709=CARTESIAN_POINT ( 'NONE',  ( -198.0356074513804572, 39.15871834505956173, -39.15871834505865223 ) ) ;
#9744=PRODUCT_DEFINITION_SHAPE ( 'NONE', 'NONE',  #25182 ) ;
#9779=CARTESIAN_POINT ( 'NONE',  ( 200.0000000000001137, 18.84395317400427317, -2.458366139920278304 ) ) ;
#9780=CARTESIAN_POINT ( 'NONE',  ( 199.9999999999999432, -11.82405030923947997, -14.88174658256811256 ) ) ;
#9790=CARTESIAN_POINT ( 'NONE',  ( 200.0000000000000000, -13.44239485489230290, 13.44239485489200803 ) ) ;
#9791=CARTESIAN_POINT ( 'NONE',  ( 136.1360204305621551, 3.511608612530062512, 53.05693388239318864 ) ) ;
#9794=CARTESIAN_POINT ( 'NONE',  ( 163.1118516004056573, -19.27778845538787422, 19.27778845538743724 ) ) ;
#9804=CARTESIAN_POINT ( 'NONE',  ( 199.9999999999998295, -18.94756416210704941, 1.560766781390804381 ) ) ;
#9807=EDGE_CURVE ( 'NONE', #21343, #15869, #4384, .T. ) ;
#9810=CARTESIAN_POINT ( 'NONE',  ( 199.0054512189284424, 16.16316501604694622, -11.77153054567511425 ) ) ;
#9837=CARTESIAN_POINT ( 'NONE',  ( 200.0000000000000000, 18.87777001997802628, 2.191952217553565507 ) ) ;
#9844=CARTESIAN_POINT ( 'NONE',  ( 4.995406935893290878, 39.06748935135239265, -39.06748935135144762 ) ) ;
#9870=CARTESIAN_POINT ( 'NONE',  ( 199.9999999999999147, 16.69452638465319083, -9.073307399871135104 ) ) ;
#9876=CARTESIAN_POINT ( 'NONE',  ( 199.0097900131551114, -3.258944298918965199, -19.73026277452668609 ) ) ;
#9885=CARTESIAN_POINT ( 'NONE',  ( 199.0157948715101668, 14.36126147255820484, 13.92041998760680066 ) ) ;
#9903=DIRECTION ( 'NONE',  ( 0.000000000000000000, -1.000000000000000000, 0.000000000000000000 ) ) ;
#9910=CARTESIAN_POINT ( 'NONE',  ( 199.9999999999996874, 18.57765777299087873, -3.990914148134230288 ) ) ;
#9911=CARTESIAN_POINT ( 'NONE',  ( 199.9999999999998863, -15.63633292130449703, 10.81305911573160472 ) ) ;
#9921=CARTESIAN_POINT ( 'NONE',  ( 199.0263117993877131, -12.25726513653892447, 15.86500832304671427 ) ) ;
#9922=CARTESIAN_POINT ( 'NONE',  ( -91.56559293963834989, -16.03295912088659492, -40.53558337403696044 ) ) ;
#9935=CARTESIAN_POINT ( 'NONE',  ( 199.9999999999994031, -18.37269623729978107, -4.912321869774860517 ) ) ;
#9938=CARTESIAN_POINT ( 'NONE',  ( 199.0186803405091780, -17.32754287553631301, -9.995805879000721816 ) ) ;
#9941=EDGE_CURVE ( 'NONE', #21338, #21343, #19902, .T. ) ;
#9966=EDGE_LOOP ( 'NONE', ( #16815, #5514, #23671, #8331 ) ) ;
#9970=CARTESIAN_POINT ( 'NONE',  ( 200.0000000000000284, 12.51656570147539327, 14.30544205704861760 ) ) ;
#9976=CARTESIAN_POINT ( 'NONE',  ( 151.7948205124836250, 4.785054706301759886, -4.785054706301612448 ) ) ;
#9977=CARTESIAN_POINT ( 'NONE',  ( 199.0232347278000873, 0.3099713519423794028, 20.00382596759649800 ) ) ;
#10003=CARTESIAN_POINT ( 'NONE',  ( 199.9999999999999432, 18.40126832602490481, -4.753217589480088989 ) ) ;
#10009=CARTESIAN_POINT ( 'NONE',  ( 199.0099327931564233, -3.581876008808642098, -19.67427284064525139 ) ) ;
#10014=CARTESIAN_POINT ( 'NONE',  ( 199.9999999999998863, -16.91159699891635171, 8.687942971654136315 ) ) ;
#10017=CARTESIAN_POINT ( 'NONE',  ( 199.0225339954500328, 2.108197227390415929, 19.89250884296043864 ) ) ;
#10047=CARTESIAN_POINT ( 'NONE',  ( 199.9999999999997442, 15.07190321012488887, 11.58049570127731798 ) ) ;
#10048=CARTESIAN_POINT ( 'NONE',  ( 199.9999999999999716, -17.84994651634582397, 6.552042691338741953 ) ) ;
#10057=CARTESIAN_POINT ( 'NONE',  ( 199.0197853254965707, 8.008002382618863990, 18.32953931431698535 ) ) ;
#10059=CARTESIAN_POINT ( 'NONE',  ( 14.38125909742180397, 67.30136555898270956, -10.73282306405792319 ) ) ;
#10072=CARTESIAN_POINT ( 'NONE',  ( 200.0000000000003411, -18.28334586770733594, 5.214203034309022655 ) ) ;
#10075=CARTESIAN_POINT ( 'NONE',  ( 199.0080442515877905, 1.130919702028742257, -19.96471691786700120 ) ) ;
#10103=CARTESIAN_POINT ( 'NONE',  ( 199.9999999999998295, 8.812783067309094776, 16.84096882534935702 ) ) ;
#10110=CARTESIAN_POINT ( 'NONE',  ( -192.9588430854690273, 10.23066800229588758, -66.79921049721882298 ) ) ;
#10111=CARTESIAN_POINT ( 'NONE',  ( 199.0263771359574889, -13.68429728450633753, 14.60718570525551563 ) ) ;
#10136=CARTESIAN_POINT ( 'NONE',  ( 199.9999999999999432, 17.05889967449044775, -8.389830104632190810 ) ) ;
#10143=CARTESIAN_POINT ( 'NONE',  ( 199.0120775374408311, -7.960707704260069129, -18.34818886981279462 ) ) ;
#10155=CARTESIAN_POINT ( 'NONE',  ( 199.0228608363770206, 1.289830063590766907, 19.96444201077071057 ) ) ;
#10180=CARTESIAN_POINT ( 'NONE',  ( 199.9999999999998579, 17.78360892267977178, 6.705045715290576247 ) ) ;
#10181=CARTESIAN_POINT ( 'NONE',  ( 199.9999999999999716, -17.44173617362904949, 7.567414129180135340 ) ) ;
#10190=CARTESIAN_POINT ( 'NONE',  ( 199.0199705922642295, 7.656373194246554270, 18.47861116135505100 ) ) ;
#10192=CARTESIAN_POINT ( 'NONE',  ( -86.96347745069644475, 12.89780903124419353, -12.89780903124389333 ) ) ;
#10194=CARTESIAN_POINT ( 'NONE',  ( 14.38125909742180397, 67.30136555898270956, -10.73282306405792319 ) ) ;
#10205=CARTESIAN_POINT ( 'NONE',  ( 199.9999999999998863, -18.99932777274695539, 0.6272729670678898195 ) ) ;
#10209=CARTESIAN_POINT ( 'NONE',  ( 199.0127284201194300, -9.139505923766694906, -17.79079187713806220 ) ) ;
#10236=CARTESIAN_POINT ( 'NONE',  ( 200.0000000000000284, 17.23849352212496910, 7.999418879479941680 ) ) ;
#10242=CARTESIAN_POINT ( 'NONE',  ( -280.0000000000000568, -14.14213562373049449, -42.42640687119305198 ) ) ;
#10243=DIRECTION ( 'NONE',  ( 0.000000000000000000, -1.000000000000000000, 0.000000000000000000 ) ) ;
#10268=( LENGTH_UNIT ( ) NAMED_UNIT ( * ) SI_UNIT ( .MILLI., .METRE. ) );
#10272=CARTESIAN_POINT ( 'NONE',  ( 199.9999999999999432, 9.226325135675029543, 16.62006860685476184 ) ) ;
#10278=CARTESIAN_POINT ( 'NONE',  ( 199.0073291892102247, 3.255542347464756681, -19.72957075196997323 ) ) ;
#10287=CARTESIAN_POINT ( 'NONE',  ( 199.0210534451952924, 5.480999013853959489, 19.23967134089702569 ) ) ;
#10315=CARTESIAN_POINT ( 'NONE',  ( 200.0000000000001137, 18.27430636540404407, -5.205727087885991367 ) ) ;
#10316=CARTESIAN_POINT ( 'NONE',  ( 199.9999999999999716, -16.47313602895343365, 9.508414938895898061 ) ) ;
#10319=DIRECTION ( 'NONE',  ( -1.000000000000000000, -1.836970198721030181E-16, -1.232595164407830946E-32 ) ) ;
#10325=CARTESIAN_POINT ( 'NONE',  ( 199.0254843815459651, -7.164921656906469316, 18.67865466993989898 ) ) ;
#10326=CARTESIAN_POINT ( 'NONE',  ( -162.0762913951020892, 29.48230308784799902, -29.48230308784730980 ) ) ;
#10328=CARTESIAN_POINT ( 'NONE',  ( -280.0000000000000568, 42.42640687119265408, 14.14213562373147504 ) ) ;
#10339=CARTESIAN_POINT ( 'NONE',  ( 199.0095093599360894, -2.612260778589423182, -19.82812366214328748 ) ) ;
#10365=CARTESIAN_POINT ( 'NONE',  ( 200.0000000000002842, 4.912815075579886503, -18.35721014059308942 ) ) ;
#10372=CARTESIAN_POINT ( 'NONE',  ( 192.4448373802101173, -42.42640687122053578, -14.14213562370360577 ) ) ;
#10373=CARTESIAN_POINT ( 'NONE',  ( 199.0258313909553749, -8.851116586292111066, 17.94317422212728630 ) ) ;
#10396=CARTESIAN_POINT ( 'NONE',  ( 199.9999999999999432, 14.88226939975712604, 11.82339673543941494 ) ) ;
#10403=CARTESIAN_POINT ( 'NONE',  ( 199.0117582043400830, -7.359043231587310885, -18.59750019459799120 ) ) ;
#10412=CARTESIAN_POINT ( 'NONE',  ( 199.0056892241198625, 17.33029760820262410, -9.978133259584877734 ) ) ;
#10441=CARTESIAN_POINT ( 'NONE',  ( 200.0000000000000568, 2.630809070280605511, -18.81871160794394982 ) ) ;
#10445=CARTESIAN_POINT ( 'NONE',  ( 199.9999999999999147, 11.06273067492490547, -15.45041022988906931 ) ) ;
#10456=CARTESIAN_POINT ( 'NONE',  ( 151.7948205124836534, 33.06932595376333239, 23.49921654116065284 ) ) ;
#10458=CARTESIAN_POINT ( 'NONE',  ( -86.96347745069644475, 12.89780903124349898, 43.67073346367994446 ) ) ;
#10473=CARTESIAN_POINT ( 'NONE',  ( 199.0099327931564233, -3.581876008808642098, -19.67427284064525139 ) ) ;
#10500=CARTESIAN_POINT ( 'NONE',  ( 199.9999999999997726, 3.400090818600995934, -18.69490476363523612 ) ) ;
#10506=CARTESIAN_POINT ( 'NONE',  ( -100.7734535825088358, -16.03295912088728770, 16.03295912088687913 ) ) ;
#10507=CARTESIAN_POINT ( 'NONE',  ( 199.0246859915949642, -4.071254240408448410, 19.58630271169732140 ) ) ;
#10518=CARTESIAN_POINT ( 'NONE',  ( 199.0260893535204048, -10.43036187021208860, 17.07141274968551059 ) ) ;
#10531=CARTESIAN_POINT ( 'NONE',  ( 199.9999999999999147, -10.44179787682348781, 15.88662230291588706 ) ) ;
#10538=CARTESIAN_POINT ( 'NONE',  ( 199.0166470710653925, -15.03895783737594805, -13.18902814565699266 ) ) ;
#10549=CARTESIAN_POINT ( 'NONE',  ( 199.0070393743141892, 19.55016766319115007, -4.199986046643529924 ) ) ;
#10562=CARTESIAN_POINT ( 'NONE',  ( 199.0142503478488720, -11.66167433960233168, -16.26558534365442910 ) ) ;
#10574=CARTESIAN_POINT ( 'NONE',  ( 199.9999999999998295, 14.29413690760092592, -12.53266873553815053 ) ) ;
#10575=CARTESIAN_POINT ( 'NONE',  ( 199.9999999999999147, -1.558418107136771757, -18.94039843610738671 ) ) ;
#10587=CARTESIAN_POINT ( 'NONE',  ( -105.3755690713226585, -43.67073346367964604, -12.89780903124457545 ) ) ;
#10589=CARTESIAN_POINT ( 'NONE',  ( -135.8532207217289738, 50.09629031063956006, 6.472252184284782217 ) ) ;
#10604=CARTESIAN_POINT ( 'NONE',  ( 200.0000000000003411, -11.08347333911627963, 15.44584840147742355 ) ) ;
#10620=ADVANCED_FACE ( 'NONE', ( #5335 ), #21437, .F. ) ;
#10623=PRODUCT ( 'Rotor', 'Rotor', '', ( #22078 ) ) ;
#10640=CARTESIAN_POINT ( 'NONE',  ( 200.0000000000002842, 11.06692676694369304, -15.45668394874709506 ) ) ;
#10643=CARTESIAN_POINT ( 'NONE',  ( -213.1075012329537230, -18.58567234101102272, -37.98287015391260013 ) ) ;
#10644=CARTESIAN_POINT ( 'NONE',  ( 199.0087145623001277, 19.98798542585446469, 0.6659850717246563745 ) ) ;
#10670=CARTESIAN_POINT ( 'NONE',  ( 200.0000000000000000, -13.44239485489230290, 13.44239485489200803 ) ) ;
#10676=CARTESIAN_POINT ( 'NONE',  ( 199.0174211633917878, -15.97280307358279039, -12.03849830368706009 ) ) ;
#10689=CARTESIAN_POINT ( 'NONE',  ( 199.0124915487878923, 17.99959093953023270, 8.716253503037693307 ) ) ;
#10705=CARTESIAN_POINT ( 'NONE',  ( 199.0155016027679551, -13.51399019912108557, -14.74480745368398971 ) ) ;
#10716=CARTESIAN_POINT ( 'NONE',  ( 199.9999999999997726, 3.400090818600995934, -18.69490476363523612 ) ) ;
#10726=CARTESIAN_POINT ( 'NONE',  ( 199.0129076123475045, 17.63563449655302051, 9.445111419240257433 ) ) ;
#10727=CARTESIAN_POINT ( 'NONE',  ( -198.0356074513804572, 10.87444709759730088, -10.87444709759707173 ) ) ;
#10742=CARTESIAN_POINT ( 'NONE',  ( 199.0258314272957421, -17.94308652430182605, 8.851303907023687856 ) ) ;
#10768=CARTESIAN_POINT ( 'NONE',  ( 199.9999999999998010, 17.44192585402499418, -7.542491233669909256 ) ) ;
#10772=CARTESIAN_POINT ( 'NONE',  ( 199.9999999999999432, -14.14213562373115884, 14.14213562373085153 ) ) ;
#10773=CARTESIAN_POINT ( 'NONE',  ( 199.0198237862232133, 7.937771492746675150, 18.36232769351375538 ) ) ;
#10803=CARTESIAN_POINT ( 'NONE',  ( 199.9999999999999432, -4.478796266106241042, 18.47916794701787069 ) ) ;
#10806=ORIENTED_EDGE ( 'NONE', *, *, #26161, .T. ) ;
#10809=CARTESIAN_POINT ( 'NONE',  ( 199.0242480509055270, -19.84286657041863933, 2.617213520271152394 ) ) ;
#10820=CARTESIAN_POINT ( 'NONE',  ( 199.0073354103614918, 19.73522450985164411, -3.233483297802316692 ) ) ;
#10834=CARTESIAN_POINT ( 'NONE',  ( 199.0053898862218205, 12.24380588499195888, -15.86248857793228595 ) ) ;
#10844=CARTESIAN_POINT ( 'NONE',  ( 199.9999999999998579, 7.403094706059546226, -17.49952075364730675 ) ) ;
#10845=CARTESIAN_POINT ( 'NONE',  ( 199.9999999999999147, 8.817827506411962446, -16.83089631069017145 ) ) ;
#10854=CARTESIAN_POINT ( 'NONE',  ( 199.0081480328640566, 19.97905789705941260, -0.8430309673498267431 ) ) ;
#10855=CARTESIAN_POINT ( 'NONE',  ( -259.2033419157646676, -6.730120644403663199, 6.730120644403451813 ) ) ;
#10875=CARTESIAN_POINT ( 'NONE',  ( 199.0232879746372134, -20.00360196692749071, -0.1645009869758431997 ) ) ;
#10905=CARTESIAN_POINT ( 'NONE',  ( 200.0000000000001421, 17.31676413174603013, -7.825505819403215213 ) ) ;
#10908=CARTESIAN_POINT ( 'NONE',  ( -238.4067589809705794, 0.6820004457912851592, -0.6820004457913123597 ) ) ;
#10909=CARTESIAN_POINT ( 'NONE',  ( 199.0120006491917479, 18.40818734026414560, 7.815811290271758693 ) ) ;
#10937=CARTESIAN_POINT ( 'NONE',  ( 199.9999999999999147, -4.931750674013845703, 18.35953736552815130 ) ) ;
#10943=CARTESIAN_POINT ( 'NONE',  ( 199.0161314855084527, -14.37392100214799839, -13.91043101682956973 ) ) ;
#10956=CARTESIAN_POINT ( 'NONE',  ( 199.0054512189284424, 16.16316501604694622, -11.77153054567511425 ) ) ;
#10971=CARTESIAN_POINT ( 'NONE',  ( 199.0084482301557216, 0.03073351504823504388, -19.99623419276333536 ) ) ;
#10982=CARTESIAN_POINT ( 'NONE',  ( 199.9999999999998863, -4.322767242657778120, -18.50495320732392557 ) ) ;
#10983=CARTESIAN_POINT ( 'NONE',  ( 199.9999999999999716, -5.827982453606887603, -18.08981252677385498 ) ) ;
#10991=CARTESIAN_POINT ( 'NONE',  ( 199.0053897493126556, 15.86173083671449113, -12.24509968457356202 ) ) ;
#10992=CARTESIAN_POINT ( 'NONE',  ( -100.7734535825088358, -16.03295912088728770, 16.03295912088687913 ) ) ;
#11005=CARTESIAN_POINT ( 'NONE',  ( 199.0234090143162859, -20.00365258984362882, 0.1656111763342176801 ) ) ;
#11031=CARTESIAN_POINT ( 'NONE',  ( 199.9999999999998579, -10.30558286630674658, -15.96802547070553047 ) ) ;
#11035=CARTESIAN_POINT ( 'NONE',  ( 199.0128224874292471, 17.70345943908711561, 9.303337553156843853 ) ) ;
#11050=CARTESIAN_POINT ( 'NONE',  ( -56.48582580120559982, 21.81201906317729922, 34.75652343174635917 ) ) ;
#11058=CARTESIAN_POINT ( 'NONE',  ( -192.9588430854689989, 10.23066800230756712, -10.23066800230735396 ) ) ;
#11066=CARTESIAN_POINT ( 'NONE',  ( 199.0208257245452899, -19.09599194444923143, -5.955353076589812389 ) ) ;
#11092=CARTESIAN_POINT ( 'NONE',  ( 199.0119170695921582, -7.658365714851820272, -18.47347012762973151 ) ) ;
#11102=CARTESIAN_POINT ( 'NONE',  ( 200.0000000000000000, -10.04040541317802315, -16.13598245992451297 ) ) ;
#11113=EDGE_CURVE ( 'NONE', #21343, #21338, #6323, .T. ) ;
#11116=CARTESIAN_POINT ( 'NONE',  ( -238.4067589809705794, 0.6820004457912851592, -0.6820004457913123597 ) ) ;
#11130=CARTESIAN_POINT ( 'NONE',  ( 199.0053211801402426, 14.13499912481545451, -14.14174623454970536 ) ) ;
#11131=CARTESIAN_POINT ( 'NONE',  ( 199.0228518427889242, -19.96294788386713037, -1.312843269464072815 ) ) ;
#11154=CARTESIAN_POINT ( 'NONE',  ( 199.9999999999999147, 1.697088945475840660, -18.92594139730135439 ) ) ;
#11157=CARTESIAN_POINT ( 'NONE',  ( 199.0127395736742244, 17.77917978336349236, 9.157720830221606434 ) ) ;
#11171=CARTESIAN_POINT ( 'NONE',  ( -105.3755690713226727, -15.38646221621807619, 15.38646221621768362 ) ) ;
#11185=CARTESIAN_POINT ( 'NONE',  ( 199.9999999999997726, -8.411091645968788555, 17.05096182211362432 ) ) ;
#11187=ADVANCED_FACE ( 'NONE', ( #4470, #22565 ), #12436, .T. ) ;
#11192=ADVANCED_BREP_SHAPE_REPRESENTATION ( '', ( #26080, #21058 ), #20184 ) ;
#11216=CARTESIAN_POINT ( 'NONE',  ( 199.0233417977821091, -20.00361827599568798, -0.01770272352667627211 ) ) ;
#11226=CARTESIAN_POINT ( 'NONE',  ( 199.9999999999998579, -18.00099009291985297, -6.105420735363839668 ) ) ;
#11251=CARTESIAN_POINT ( 'NONE',  ( 200.0000000000000000, 2.003163845861910097, 18.90332168644373567 ) ) ;
#11253=CARTESIAN_POINT ( 'NONE',  ( 200.0000000000000000, -13.44239485489230290, 13.44239485489200803 ) ) ;
#11278=CARTESIAN_POINT ( 'NONE',  ( 200.0000000000005116, -0.6320235832414241584, -19.00127953747481868 ) ) ;
#11282=CARTESIAN_POINT ( 'NONE',  ( 199.0067627483201989, 19.31843298438769807, -5.161535144790875940 ) ) ;
#11311=CARTESIAN_POINT ( 'NONE',  ( 199.9999999999998863, -7.850736592177782747, 17.31604939001003274 ) ) ;
#11338=ORIENTED_EDGE ( 'NONE', *, *, #19215, .T. ) ;
#11340=CARTESIAN_POINT ( 'NONE',  ( 199.0233350887612289, -20.00359049402684875, -0.03597354547537223030 ) ) ;
#11350=CARTESIAN_POINT ( 'NONE',  ( 199.9999999999999147, -14.49496992596536771, -12.29673964441684042 ) ) ;
#11372=CARTESIAN_POINT ( 'NONE',  ( 199.9999999999999716, -3.868950841772955673, 18.61236034055575317 ) ) ;
#11395=CARTESIAN_POINT ( 'NONE',  ( 199.9999999999997726, -2.174764995058875439, -18.87968408895515182 ) ) ;
#11399=CARTESIAN_POINT ( 'NONE',  ( 199.0077026597514021, 2.114100997916472657, -19.88449140175694296 ) ) ;
#11431=CARTESIAN_POINT ( 'NONE',  ( 199.0263730241462099, -14.60190056250242030, 13.67829565473005715 ) ) ;
#11456=( BOUNDED_CURVE ( )  B_SPLINE_CURVE ( 3, ( #3023, #5399, #11130, #26299 ),
 .UNSPECIFIED., .F., .T. ) 
 B_SPLINE_CURVE_WITH_KNOTS ( ( 4, 4 ),
 ( 0.4999406519327141418, 0.5000000000000000000 ),
 .UNSPECIFIED. ) 
 CURVE ( )  GEOMETRIC_REPRESENTATION_ITEM ( )  RATIONAL_B_SPLINE_CURVE ( ( 1.000000000000000000, 0.9998807446028390444, 0.9997615105384527467, 0.9996422978068409959 ) ) 
 REPRESENTATION_ITEM ( '' )  );
#11460=CARTESIAN_POINT ( 'NONE',  ( 199.0233445383804565, -20.00362565020445871, -0.01023483319826397862 ) ) ;
#11470=CARTESIAN_POINT ( 'NONE',  ( 199.9999999999999147, -18.99336422956244874, -0.7807574862979690389 ) ) ;
#11499=CARTESIAN_POINT ( 'NONE',  ( 200.0000000000000284, -9.508146755684434126, 16.46234680784547777 ) ) ;
#11524=CARTESIAN_POINT ( 'NONE',  ( 199.9999999999999147, -10.43683117453143261, -15.88259547814976180 ) ) ;
#11527=CARTESIAN_POINT ( 'NONE',  ( 199.0056892241198625, 17.33029760820262410, -9.978133259584877734 ) ) ;
#11557=CARTESIAN_POINT ( 'NONE',  ( 199.9999999999997726, -5.383989893674753446, 18.23209102328170061 ) ) ;
#11589=CARTESIAN_POINT ( 'NONE',  ( 199.0227794283635205, -19.94987460103941501, -1.494179565802910670 ) ) ;
#11602=CARTESIAN_POINT ( 'NONE',  ( 200.0000000000000853, -8.685123034760072969, -16.90575535186691880 ) ) ;
#11629=CARTESIAN_POINT ( 'NONE',  ( 199.9999999999998863, 12.86276811643300810, 13.99220397845184749 ) ) ;
#11641=CARTESIAN_POINT ( 'NONE',  ( 136.1360204305621266, -24.77266263493151044, 24.77266263493093135 ) ) ;
#11654=CARTESIAN_POINT ( 'NONE',  ( 200.0000000000001705, -18.10265802883496278, 5.810802590798905598 ) ) ;
#11659=CARTESIAN_POINT ( 'NONE',  ( 199.0064300168743898, 6.416848550863170964, -18.94043562797172697 ) ) ;
#11677=CARTESIAN_POINT ( 'NONE',  ( 191.7962200090128988, -14.19927417784172974, 14.19927417784142243 ) ) ;
#11688=CARTESIAN_POINT ( 'NONE',  ( 199.0261122283987731, -17.00127104892409591, 10.56324628376440877 ) ) ;
#11695=CARTESIAN_POINT ( 'NONE',  ( -208.1127848780265026, 38.89260858015777700, -38.89260858015687461 ) ) ;
#11699=VECTOR ( 'NONE', #21699, 1000.000000000000000 ) ;
#11729=CARTESIAN_POINT ( 'NONE',  ( 199.0255884649229756, -18.48832673850237285, 7.640083164573010954 ) ) ;
#11737=CARTESIAN_POINT ( 'NONE',  ( 57.59792236341147031, 26.56190807104720975, -26.56190807104655249 ) ) ;
#11739=CARTESIAN_POINT ( 'NONE',  ( 200.0000000000000853, -18.58433719308212773, 4.010382776060092525 ) ) ;
#11770=CARTESIAN_POINT ( 'NONE',  ( 200.0000000000001421, 18.96284454896564142, 1.255519873078760229 ) ) ;
#11771=CARTESIAN_POINT ( 'NONE',  ( 199.9999999999999432, -9.506243415956056708, -16.45614580735059107 ) ) ;
#11783=CARTESIAN_POINT ( 'NONE',  ( 170.2234770963711128, -17.36149277827010096, 17.36149277826970660 ) ) ;
#11786=CARTESIAN_POINT ( 'NONE',  ( 19.06497207195980792, 10.03556273973447155, -10.03556273973422286 ) ) ;
#11799=CARTESIAN_POINT ( 'NONE',  ( 199.0069392139017168, 4.538005534962026744, -19.47646040276416457 ) ) ;
#11827=CARTESIAN_POINT ( 'NONE',  ( 199.9999999999998863, 18.74710533595338546, 3.118879735276928855 ) ) ;
#11833=CARTESIAN_POINT ( 'NONE',  ( -259.2033419157646676, -6.730120644402966867, -49.83842185052038332 ) ) ;
#11834=FACE_OUTER_BOUND ( 'NONE', #23213, .T. ) ;
#11860=CARTESIAN_POINT ( 'NONE',  ( 199.9999999999999432, 11.06651829421018896, 15.46448801036256349 ) ) ;
#11866=CARTESIAN_POINT ( 'NONE',  ( 199.0069392139017168, 4.538005534962026744, -19.47646040276416457 ) ) ;
#11875=CARTESIAN_POINT ( 'NONE',  ( 199.0202951899208017, 7.027923415129357032, 18.72965638665138144 ) ) ;
#11904=CARTESIAN_POINT ( 'NONE',  ( 199.9999999999996874, 18.36026428565764945, 4.938082948735277533 ) ) ;
#11907=CARTESIAN_POINT ( 'NONE',  ( 199.9999999999999147, -18.99732930369138728, -0.7780015511921255511 ) ) ;
#11918=CARTESIAN_POINT ( 'NONE',  ( 199.0227866802457584, 1.475801328052707806, 19.95124150608079105 ) ) ;
#11919=CARTESIAN_POINT ( 'NONE',  ( -280.0000000000000568, 42.42640687119265408, 14.14213562373147504 ) ) ;
#11930=CARTESIAN_POINT ( 'NONE',  ( 199.9999999999998579, -17.31468161508541570, -7.846489601088847188 ) ) ;
#11933=CARTESIAN_POINT ( 'NONE',  ( 199.0176767632675023, -16.26464645690579758, -11.64139296301337190 ) ) ;
#11963=CARTESIAN_POINT ( 'NONE',  ( 200.0000000000001137, 4.308913765035643273, 18.51575813813059668 ) ) ;
#11970=CARTESIAN_POINT ( 'NONE',  ( -100.7734535825088358, 12.25131212657497848, -12.25131212657469604 ) ) ;
#11971=CARTESIAN_POINT ( 'NONE',  ( 199.0261966595921592, -11.26051109717869458, 16.53566845662597729 ) ) ;
#11997=CARTESIAN_POINT ( 'NONE',  ( 199.9999999999999716, 16.45620519018019579, 9.525122676133902289 ) ) ;
#12004=CARTESIAN_POINT ( 'NONE',  ( 199.0073806320087613, 3.093635517344801578, -19.75563546371214230 ) ) ;
#12011=CARTESIAN_POINT ( 'NONE',  ( 199.9999999999999147, -17.05087848619496782, 8.411269650559694000 ) ) ;
#12014=CARTESIAN_POINT ( 'NONE',  ( 199.0166590359707754, 13.17187519532568984, 15.05399639075651130 ) ) ;
#12038=CARTESIAN_POINT ( 'NONE',  ( 199.9999999999998295, 13.96930097052764097, 12.88701297307445159 ) ) ;
#12039=CARTESIAN_POINT ( 'NONE',  ( 200.0000000000000284, -15.63578675875477941, -10.80997969227835043 ) ) ;
#12048=CARTESIAN_POINT ( 'NONE',  ( 199.0248586838703773, -4.674415065593815477, 19.46161178335769293 ) ) ;
#12050=CARTESIAN_POINT ( 'NONE',  ( 0.2972598230769907257, 66.70487387989869887, -10.13633138497392494 ) ) ;
#12065=CARTESIAN_POINT ( 'NONE',  ( 199.9999999999996874, -18.99916535394237727, -0.6249076428296399532 ) ) ;
#12068=CARTESIAN_POINT ( 'NONE',  ( 199.0134806391063194, -10.42534412885540185, -17.06722571675988931 ) ) ;
#12096=CARTESIAN_POINT ( 'NONE',  ( 199.9999999999996589, 6.678198862535981384, 17.79829383751451388 ) ) ;
#12102=CARTESIAN_POINT ( 'NONE',  ( 91.82158438592158234, -12.16597498399995203, -44.40256751092347542 ) ) ;
#12103=CARTESIAN_POINT ( 'NONE',  ( 199.0219179450577371, 3.573952992290374109, 19.68174087806957573 ) ) ;
#12131=CARTESIAN_POINT ( 'NONE',  ( 199.9999999999999432, 13.20576333637327693, 13.67145050352531399 ) ) ;
#12137=CARTESIAN_POINT ( 'NONE',  ( 199.0127284201194300, -9.139505923766694906, -17.79079187713806220 ) ) ;
#12142=CARTESIAN_POINT ( 'NONE',  ( 199.9999999999999716, -17.31617203886849410, 7.850475485701642775 ) ) ;
#12147=CARTESIAN_POINT ( 'NONE',  ( 199.0235930299571123, -0.6679962965002699260, 20.00321896753086648 ) ) ;
#12175=CARTESIAN_POINT ( 'NONE',  ( 200.0000000000002558, 14.28373528157942829, 12.54030857537068755 ) ) ;
#12176=CARTESIAN_POINT ( 'NONE',  ( 199.9999999999998863, -13.00209652640642943, -13.87527625954625954 ) ) ;
#12185=CARTESIAN_POINT ( 'NONE',  ( 199.0263771353515949, -14.14574067859894413, 14.14574067859863682 ) ) ;
#12186=CARTESIAN_POINT ( 'NONE',  ( 163.1118516004056573, 9.006482792069759213, -9.006482792069505194 ) ) ;
#12188=CARTESIAN_POINT ( 'NONE',  ( 151.7948205124836534, 4.785054706297857230, 51.78348778862544322 ) ) ;
#12198=CARTESIAN_POINT ( 'NONE',  ( 199.9999999999998295, -19.00894346483091724, 0.1575548292166454312 ) ) ;
#12202=CARTESIAN_POINT ( 'NONE',  ( 199.0116000645839449, -7.055149577161559549, -18.71482085160166875 ) ) ;
#12228=CARTESIAN_POINT ( 'NONE',  ( 199.9999999999998863, 12.86276811643300810, 13.99220397845184749 ) ) ;
#12235=CARTESIAN_POINT ( 'NONE',  ( 170.2234770963711128, 10.92277846919216522, -10.92277846919186501 ) ) ;
#12236=CARTESIAN_POINT ( 'NONE',  ( 199.0260481038674811, -10.14773143618404383, 17.24088832081764622 ) ) ;
#12263=CARTESIAN_POINT ( 'NONE',  ( 200.0000000000000000, 13.86690804110605590, 13.01115396687990433 ) ) ;
#12269=CARTESIAN_POINT ( 'NONE',  ( 199.0089689370622352, -1.315408825438062257, -19.96384840600867960 ) ) ;
#12274=CARTESIAN_POINT ( 'NONE',  ( 199.9999999999996874, -18.85616045826023779, 2.487226269395955480 ) ) ;
#12278=CARTESIAN_POINT ( 'NONE',  ( 199.0191753821509622, 9.128090787448098098, 17.79799345705162139 ) ) ;
#12297=CARTESIAN_POINT ( 'NONE',  ( -265.0000000000000000, -10.00000000000004796, -6.532754371361504014E-30 ) ) ;
#12300=CARTESIAN_POINT ( 'NONE',  ( 199.9999999999998295, 18.60987205011830881, -3.837998380785754726 ) ) ;
#12301=CARTESIAN_POINT ( 'NONE',  ( 199.9999999999998863, -19.00899821966885028, 0.6240211523505900804 ) ) ;
#12311=CARTESIAN_POINT ( 'NONE',  ( 199.0164216790778084, 13.51997225171141892, 14.76318892796115811 ) ) ;
#12313=CARTESIAN_POINT ( 'NONE',  ( -162.0762913951020892, 1.198031840456041497, -57.76657433537918251 ) ) ;
#12315=CARTESIAN_POINT ( 'NONE',  ( -105.3755690713226585, 41.18208027870575449, 15.38646221621837107 ) ) ;
#12322=ORIENTED_EDGE ( 'NONE', *, *, #13513, .T. ) ;
#12327=( GEOMETRIC_REPRESENTATION_CONTEXT ( 3 ) GLOBAL_UNCERTAINTY_ASSIGNED_CONTEXT ( ( #9539 ) ) GLOBAL_UNIT_ASSIGNED_CONTEXT ( ( #1206, #15173, #5198 ) ) REPRESENTATION_CONTEXT ( 'NONE', 'WORKASPACE' ) );
#12329=CARTESIAN_POINT ( 'NONE',  ( 199.0188446093723371, -17.48804260178791736, -9.712431339257729945 ) ) ;
#12354=CARTESIAN_POINT ( 'NONE',  ( 199.9999999999996305, 11.56193655722446678, 15.09741884674619072 ) ) ;
#12360=CARTESIAN_POINT ( 'NONE',  ( 170.2234770963711128, -45.64576402573167258, -10.92277846919254891 ) ) ;
#12361=CARTESIAN_POINT ( 'NONE',  ( 199.0262408397048262, -11.66336112630027877, 16.25405011469380057 ) ) ;
#12378=CARTESIAN_POINT ( 'NONE',  ( -198.0356074513804572, 10.87444709759730088, -10.87444709759707173 ) ) ;
#12391=CARTESIAN_POINT ( 'NONE',  ( 199.9999999999998863, 17.32309309515417439, -7.829923752638988432 ) ) ;
#12397=CARTESIAN_POINT ( 'NONE',  ( 199.0132273568269170, -10.00203194272371476, -17.32088655864767190 ) ) ;
#12407=CARTESIAN_POINT ( 'NONE',  ( 199.0147602753770855, 15.66021538362855381, 12.44349737331557648 ) ) ;
#12432=CARTESIAN_POINT ( 'NONE',  ( 200.0000000000003126, 10.03286793820859835, -16.13825081434616493 ) ) ;
#12433=CARTESIAN_POINT ( 'NONE',  ( 199.9999999999999716, 6.682634084700803889, -17.78923626348730735 ) ) ;
#12436=PLANE ( 'NONE',  #13969 ) ;
#12442=CARTESIAN_POINT ( 'NONE',  ( 199.0179910436408761, 11.13570414284889409, 16.62722890173126444 ) ) ;
#12443=CARTESIAN_POINT ( 'NONE',  ( -208.1127848780264742, 10.60833733268383483, -67.17687982760675425 ) ) ;
#12446=CARTESIAN_POINT ( 'NONE',  ( -192.9588430854690273, 38.51493924976913519, 18.05360324515490333 ) ) ;
#12458=CARTESIAN_POINT ( 'NONE',  ( 199.0137359473271488, -10.84478214295758036, -16.80398351328055639 ) ) ;
#12488=CARTESIAN_POINT ( 'NONE',  ( 199.9999999999999432, 15.63063699308155030, -10.80328371702407786 ) ) ;
#12493=CARTESIAN_POINT ( 'NONE',  ( -86.96347745069644475, -15.38646221621807442, 15.38646221621768184 ) ) ;
#12494=CARTESIAN_POINT ( 'NONE',  ( 199.0238195103507053, -1.318470765087343954, 19.97100952642404437 ) ) ;
#12517=CARTESIAN_POINT ( 'NONE',  ( 199.9999999999999716, -4.021883954748531664, 18.58191672459730981 ) ) ;
#12523=CARTESIAN_POINT ( 'NONE',  ( 199.0256572979843099, -18.35487425740099354, 7.962169344204487409 ) ) ;
#12534=CARTESIAN_POINT ( 'NONE',  ( 199.0097993503064515, 19.72850438885342328, 3.281923459752313921 ) ) ;
#12550=CARTESIAN_POINT ( 'NONE',  ( 199.0081457482208691, 0.8493142590133723191, -19.97879119992165187 ) ) ;
#12563=CARTESIAN_POINT ( 'NONE',  ( 199.9999999999998863, 3.552885321105354599, -18.66644157592937248 ) ) ;
#12565=CARTESIAN_POINT ( 'NONE',  ( 199.9999999999999716, -4.928604136524651125, -18.35504861699862289 ) ) ;
#12579=CARTESIAN_POINT ( 'NONE',  ( -259.2033419157646676, -6.730120644402966867, -49.83842185052038332 ) ) ;
#12581=CARTESIAN_POINT ( 'NONE',  ( 130.8568914410475088, 4.207082182989012153, 52.36146031193425188 ) ) ;
#12595=CARTESIAN_POINT ( 'NONE',  ( 199.0239263494850093, -19.93905678827826122, 1.642264957757122890 ) ) ;
#12625=CARTESIAN_POINT ( 'NONE',  ( 199.9999999999997726, 13.87428525677396607, -12.99608892921076198 ) ) ;
#12629=CARTESIAN_POINT ( 'NONE',  ( 151.7948205124836534, -51.78348778862529400, -4.785054706299085581 ) ) ;
#12630=CARTESIAN_POINT ( 'NONE',  ( 199.0186810464772691, 9.993108295904475469, 17.32680936265314386 ) ) ;
#12657=CARTESIAN_POINT ( 'NONE',  ( 199.9999999999999716, 0.6068915371250974689, 19.00166003603166587 ) ) ;
#12663=CARTESIAN_POINT ( 'NONE',  ( 199.0183492910935286, -16.99256592298258184, -10.55490704374186883 ) ) ;
#12674=CARTESIAN_POINT ( 'NONE',  ( 199.0062091525825849, 18.60380424647159003, -7.335505861489442836 ) ) ;
#12688=CARTESIAN_POINT ( 'NONE',  ( 199.0123610602811652, -8.481086321338421996, -18.11865150390393708 ) ) ;
#12700=CARTESIAN_POINT ( 'NONE',  ( 200.0000000000001990, 8.399020763088516972, -17.04381686846133803 ) ) ;
#12701=CARTESIAN_POINT ( 'NONE',  ( 199.9999999999999432, 11.80293207093641961, -14.89258308846490664 ) ) ;
#12711=CARTESIAN_POINT ( 'NONE',  ( 184.8905102610680444, -43.07788698682556827, -13.49065550809859104 ) ) ;
#12731=CARTESIAN_POINT ( 'NONE',  ( 199.0244488197511998, -19.74721217248383809, 3.261676333419620821 ) ) ;
#12760=CARTESIAN_POINT ( 'NONE',  ( 199.9999999999995168, 19.00182775553472325, -0.6082061139381043091 ) ) ;
#12763=CARTESIAN_POINT ( 'NONE',  ( 57.59792236341147031, -1.722363176415055985, 1.722363176415024677 ) ) ;
#12764=CARTESIAN_POINT ( 'NONE',  ( 199.0140795438509826, 16.43701665320993044, 11.39707250661459348 ) ) ;
#12780=CARTESIAN_POINT ( 'NONE',  ( -238.4067589809705794, 0.6820004457912851592, -0.6820004457913123597 ) ) ;
#12789=SHAPE_REPRESENTATION_RELATIONSHIP ( 'NONE' , 'NONE' ,  #126, #11192 ) ;
#12798=CARTESIAN_POINT ( 'NONE',  ( 199.0239263494850093, -19.93905678827826122, 1.642264957757122890 ) ) ;
#12814=CARTESIAN_POINT ( 'NONE',  ( 199.0079837170424923, 19.96494570524563272, -1.290871210190707608 ) ) ;
#12843=CARTESIAN_POINT ( 'NONE',  ( 199.9999999999998295, 8.257913856993376100, -17.11264870637372226 ) ) ;
#12844=CARTESIAN_POINT ( 'NONE',  ( 199.9999999999999147, -6.992664781673325614, -17.67258180576657267 ) ) ;
#12852=CARTESIAN_POINT ( 'NONE',  ( 199.0084596282743803, 19.99626877350650744, -0.0005331044653283251991 ) ) ;
#12853=CARTESIAN_POINT ( 'NONE',  ( 151.7948205124836534, -23.49921654115981084, -33.06932595376387951 ) ) ;
#12867=CARTESIAN_POINT ( 'NONE',  ( 199.0261122283987731, -17.00127104892409591, 10.56324628376440877 ) ) ;
#12896=CARTESIAN_POINT ( 'NONE',  ( 199.9999999999997442, 18.75350838795884201, -3.072479883316599381 ) ) ;
#12899=CARTESIAN_POINT ( 'NONE',  ( -198.0356074513804572, 10.87444709759730088, -10.87444709759707173 ) ) ;
#12900=CARTESIAN_POINT ( 'NONE',  ( 199.0137418305357073, 16.79925839223816197, 10.85573510210755899 ) ) ;
#12929=CARTESIAN_POINT ( 'NONE',  ( 199.9999999999999716, 3.854709303011653709, 18.61380101728145320 ) ) ;
#12934=CARTESIAN_POINT ( 'NONE',  ( 199.0247296274817188, -19.55681251529712128, 4.220088366773818045 ) ) ;
#12945=CARTESIAN_POINT ( 'NONE',  ( 199.0263771353515949, -14.14574067859894413, 14.14574067859863682 ) ) ;
#12946=CARTESIAN_POINT ( 'NONE',  ( 199.0055119247266759, 16.54204028020789252, -11.23294693469441263 ) ) ;
#12960=CARTESIAN_POINT ( 'NONE',  ( 199.0083509329244293, 0.2901128837469029720, -19.99442784571252929 ) ) ;
#12971=CARTESIAN_POINT ( 'NONE',  ( 200.0000000000000284, -3.097043465352568248, -18.74877632928372151 ) ) ;
#12972=CARTESIAN_POINT ( 'NONE',  ( 199.9999999999999716, 0.6106555654018747115, -19.00184299465770366 ) ) ;
#12982=CARTESIAN_POINT ( 'NONE',  ( -280.0000000000000000, -14.14213562373118549, 14.14213562373078936 ) ) ;
#12999=PRODUCT_DEFINITION_FORMATION_WITH_SPECIFIED_SOURCE ( 'ANY', '', #10623, .NOT_KNOWN. ) ;
#13001=CARTESIAN_POINT ( 'NONE',  ( 199.0256572979843099, -18.35487425740099354, 7.962169344204487409 ) ) ;
#13028=CARTESIAN_POINT ( 'NONE',  ( 199.9999999999999147, 16.22794370004292830, -9.883520089760141403 ) ) ;
#13034=CARTESIAN_POINT ( 'NONE',  ( 199.0201394418415077, 7.332745681712491859, 18.61237044096938575 ) ) ;
#13049=CARTESIAN_POINT ( 'NONE',  ( 199.9999999999999432, -14.14213562373115884, 14.14213562373085153 ) ) ;
#13066=CARTESIAN_POINT ( 'NONE',  ( 199.0163032586025622, -14.59919991228128922, -13.67396374720910757 ) ) ;
#13080=CARTESIAN_POINT ( 'NONE',  ( 199.0056246187962188, 17.07746298573517052, -10.40099104823843312 ) ) ;
#13095=CARTESIAN_POINT ( 'NONE',  ( 199.0078439946754827, 1.701626800721226074, -19.92628250063794226 ) ) ;
#13104=CARTESIAN_POINT ( 'NONE',  ( 199.9999999999998579, -16.14759498898286338, -10.02975912355057453 ) ) ;
#13113=CARTESIAN_POINT ( 'NONE',  ( 199.0058908291898376, 17.93471286599577397, -8.846248472678716723 ) ) ;
#13114=CARTESIAN_POINT ( 'NONE',  ( -135.8532207217289738, -34.75652343174584757, -21.81201906317816253 ) ) ;
#13128=CARTESIAN_POINT ( 'NONE',  ( 199.9999999999999432, -11.20938440123365432, 15.35472082164171326 ) ) ;
#13155=CARTESIAN_POINT ( 'NONE',  ( 200.0000000000001705, 1.541304384858841692, -18.93928971938424155 ) ) ;
#13159=CARTESIAN_POINT ( 'NONE',  ( 199.0085879884812243, 19.99611484057871280, 0.3390174452003563710 ) ) ;
#13172=CARTESIAN_POINT ( 'NONE',  ( 199.0255290512018291, -7.361955815226616906, 18.60363316911454845 ) ) ;
#13174=CARTESIAN_POINT ( 'NONE',  ( -56.48582580120559271, -6.472252184284276844, 6.472252184284108978 ) ) ;
#13190=CARTESIAN_POINT ( 'NONE',  ( 199.9999999999995737, -5.829854758272260185, 18.09651684827149865 ) ) ;
#13219=CARTESIAN_POINT ( 'NONE',  ( 199.0199673144340409, -18.47600550957215759, -7.662649767945239887 ) ) ;
#13227=PRODUCT_DEFINITION_CONTEXT ( 'detailed design', #7971, 'design' ) ;
#13230=CARTESIAN_POINT ( 'NONE',  ( 199.9999999999997158, -17.84428681738966205, -6.548952533294360556 ) ) ;
#13255=CARTESIAN_POINT ( 'NONE',  ( 199.9999999999998579, -2.486104477534099466, 18.84865669767346574 ) ) ;
#13279=CARTESIAN_POINT ( 'NONE',  ( 199.9999999999998863, -11.82502131081330887, -14.88093782183822888 ) ) ;
#13282=CARTESIAN_POINT ( 'NONE',  ( 199.0061077845142279, 7.790749371913985755, -18.41559517569303495 ) ) ;
#13305=VERTEX_POINT ( 'NONE', #12945 ) ;
#13311=CARTESIAN_POINT ( 'NONE',  ( 199.9999999999998579, -2.486104477534099466, 18.84865669767346574 ) ) ;
#13339=CARTESIAN_POINT ( 'NONE',  ( 199.0197737566289504, -18.32000334048170487, -8.029774482221071707 ) ) ;
#13349=CARTESIAN_POINT ( 'NONE',  ( 200.0000000000000284, -19.00889450552964988, -0.1561390237190347086 ) ) ;
#13373=CARTESIAN_POINT ( 'NONE',  ( 199.9999999999995737, -5.829854758272260185, 18.09651684827149865 ) ) ;
#13401=CARTESIAN_POINT ( 'NONE',  ( 200.0000000000000284, -15.63511319855579629, -10.80754414709790190 ) ) ;
#13404=CARTESIAN_POINT ( 'NONE',  ( 199.0056860580130262, 9.997888132351027579, -17.31887563448481160 ) ) ;
#13415=AXIS2_PLACEMENT_3D ( 'NONE', #14032, #5522, #22028 ) ;
#13425=CARTESIAN_POINT ( 'NONE',  ( -162.0762913951020892, 1.198031840385732849, -1.198031840385733515 ) ) ;
#13434=CARTESIAN_POINT ( 'NONE',  ( 199.0262772983307400, -15.97594543884460450, 12.04151787815577102 ) ) ;
#13466=CARTESIAN_POINT ( 'NONE',  ( 199.0258541015842866, -17.97331862618372611, 8.883049498760815510 ) ) ;
#13476=CARTESIAN_POINT ( 'NONE',  ( 200.0000000000000284, -17.94985894478863386, -6.254032569489808679 ) ) ;
#13501=CARTESIAN_POINT ( 'NONE',  ( 200.0000000000000568, 3.396018298074437780, 18.70303282425911462 ) ) ;
#13513=EDGE_CURVE ( 'NONE', #5806, #19850, #21315, .T. ) ;
#13515=CARTESIAN_POINT ( 'NONE',  ( -213.1075012329537230, 9.698598906450543566, -9.698598906450348167 ) ) ;
#13526=CARTESIAN_POINT ( 'NONE',  ( 199.9999999999999432, -14.29115147104986860, -12.53286550942210198 ) ) ;
#13530=CARTESIAN_POINT ( 'NONE',  ( 199.0065089264240044, 19.04284699271596537, -6.106433644136123995 ) ) ;
#13548=CARTESIAN_POINT ( 'NONE',  ( -280.0000000000000000, -14.14213562373118371, 14.14213562373078936 ) ) ;
#13559=CARTESIAN_POINT ( 'NONE',  ( 200.0000000000000000, -3.101357108925543837, 18.75734389255849521 ) ) ;
#13573=CARTESIAN_POINT ( 'NONE',  ( -265.0000000000000000, -10.00000000000004796, -6.532754371361504014E-30 ) ) ;
#13598=CARTESIAN_POINT ( 'NONE',  ( 199.9999999999999147, -15.08385563027219156, -11.56407354529143205 ) ) ;
#13630=CARTESIAN_POINT ( 'NONE',  ( 199.9999999999996305, 11.56193655722446678, 15.09741884674619072 ) ) ;
#13642=CARTESIAN_POINT ( 'NONE',  ( -86.96347745069644475, 12.89780903124349898, 43.67073346367994446 ) ) ;
#13645=CARTESIAN_POINT ( 'NONE',  ( -280.0000000000000568, 14.14213562373038968, 42.42640687119305198 ) ) ;
#13656=CARTESIAN_POINT ( 'NONE',  ( 199.9999999999998010, -4.930716969832944940, -18.35446462305003834 ) ) ;
#13660=CARTESIAN_POINT ( 'NONE',  ( 199.0057329523134513, 9.713090712928652337, -17.48024697358846069 ) ) ;
#13679=CARTESIAN_POINT ( 'NONE',  ( 163.1118516004056573, -19.27778845538787422, 19.27778845538743724 ) ) ;
#13691=CARTESIAN_POINT ( 'NONE',  ( 199.9999999999997158, -10.44119114510941770, 15.88703355754643098 ) ) ;
#13696=CARTESIAN_POINT ( 'NONE',  ( 146.6084372240433993, 3.800685668858732935, -3.800685668858610367 ) ) ;
#13721=CARTESIAN_POINT ( 'NONE',  ( 199.9999999999999432, 16.46500086087206682, -9.483425485471467908 ) ) ;
#13722=CARTESIAN_POINT ( 'NONE',  ( 199.0242950697381445, -19.85973387450291128, 2.734947709465418875 ) ) ;
#13732=CARTESIAN_POINT ( 'NONE',  ( 200.0000000000000568, -14.79650836250383250, 11.93661649116771173 ) ) ;
#13758=CARTESIAN_POINT ( 'NONE',  ( 200.0000000000000568, 5.208214048020466613, 18.28294570233482119 ) ) ;
#13771=CARTESIAN_POINT ( 'NONE',  ( 14.38125909742180752, 10.73282306404735387, -10.73282306404708919 ) ) ;
#13774=CARTESIAN_POINT ( 'NONE',  ( 14.38125909742180752, 10.73282306404735387, -10.73282306404708919 ) ) ;
#13786=CARTESIAN_POINT ( 'NONE',  ( 199.0072342795740497, 19.67962538453564036, -3.556093180948044274 ) ) ;
#13792=CARTESIAN_POINT ( 'NONE',  ( 199.9999999999998863, 13.43021917686961331, -13.43983678748323918 ) ) ;
#13814=CARTESIAN_POINT ( 'NONE',  ( 199.9999999999996874, 18.36026428565764945, 4.938082948735277533 ) ) ;
#13822=CARTESIAN_POINT ( 'NONE',  ( 130.8568914410475088, -24.07718906446864793, -32.49135343045505664 ) ) ;
#13849=CARTESIAN_POINT ( 'NONE',  ( 199.9999999999999432, 19.00129205762390683, 0.6358089133326541020 ) ) ;
#13857=CARTESIAN_POINT ( 'NONE',  ( 199.0108247880216368, -5.504876786518239307, -19.22761790364454271 ) ) ;
#13863=CARTESIAN_POINT ( 'NONE',  ( 4.995406935893290878, 39.06748935135239265, -39.06748935135144762 ) ) ;
#13868=CARTESIAN_POINT ( 'NONE',  ( 199.0214920807345322, 4.534629261753806873, 19.48466678343157454 ) ) ;
#13895=CARTESIAN_POINT ( 'NONE',  ( 199.9999999999995168, 19.00182775553472325, -0.6082061139381043091 ) ) ;
#13896=CARTESIAN_POINT ( 'NONE',  ( 200.0000000000000284, -16.14727532946531241, -10.03029091962484642 ) ) ;
#13907=CARTESIAN_POINT ( 'NONE',  ( 199.0238599485892621, -1.396734769875851212, 20.00262899750501333 ) ) ;
#13908=CARTESIAN_POINT ( 'NONE',  ( -238.4067589809705794, 28.96627169325285678, 27.60227080167094726 ) ) ;
#13920=CARTESIAN_POINT ( 'NONE',  ( 199.9999999999997158, -17.84428681738966205, -6.548952533294360556 ) ) ;
#13924=CARTESIAN_POINT ( 'NONE',  ( 199.0170773700648397, -15.56690153483635264, -12.55869779031424116 ) ) ;
#13954=CARTESIAN_POINT ( 'NONE',  ( 199.9999999999996021, 18.99368777275013898, 0.6330478706754758544 ) ) ;
#13960=CARTESIAN_POINT ( 'NONE',  ( 91.82158438592158234, 16.11829626346161604, -16.11829626346121103 ) ) ;
#13969=AXIS2_PLACEMENT_3D ( 'NONE', #2210, #10319, #18426 ) ;
#13988=CARTESIAN_POINT ( 'NONE',  ( 199.9999999999999432, 12.98018377190829753, 13.88592919840850648 ) ) ;
#13995=CARTESIAN_POINT ( 'NONE',  ( 199.0080442515877905, 1.130919702028742257, -19.96471691786700120 ) ) ;
#14001=CARTESIAN_POINT ( 'NONE',  ( 199.9999999999998295, -17.79330310134281135, 6.698924172861754123 ) ) ;
#14004=CARTESIAN_POINT ( 'NONE',  ( 199.0183491629479988, 10.55513269831597079, 16.99244513920028510 ) ) ;
#14032=CARTESIAN_POINT ( 'NONE',  ( 199.9999999999999432, -2.560943207453569512E-14, 6.234883604895477860E-14 ) ) ;
#14033=CARTESIAN_POINT ( 'NONE',  ( 199.9999999999998010, 17.44192585402499418, -7.542491233669909256 ) ) ;
#14034=CARTESIAN_POINT ( 'NONE',  ( 199.9999999999999716, -16.46561772086350217, -9.499012046328999759 ) ) ;
#14043=CARTESIAN_POINT ( 'NONE',  ( 199.0233509355391277, -0.007210440545907509553, 20.00363007596296328 ) ) ;
#14044=CARTESIAN_POINT ( 'NONE',  ( -105.3755690713226727, 12.89780903124418998, -12.89780903124389155 ) ) ;
#14060=CARTESIAN_POINT ( 'NONE',  ( 199.9999999999998010, -18.94725682776174835, -1.557189005449375330 ) ) ;
#14063=CARTESIAN_POINT ( 'NONE',  ( 199.0196534518890701, -18.22073438007316071, -8.257363271777977687 ) ) ;
#14090=CARTESIAN_POINT ( 'NONE',  ( 199.9999999999998010, 13.53697630789494255, 13.34066885590318030 ) ) ;
#14098=CARTESIAN_POINT ( 'NONE',  ( -238.4067589809705794, 28.96627169325354956, -28.96627169325289231 ) ) ;
#14099=CARTESIAN_POINT ( 'NONE',  ( 199.0222638060928375, 2.763249014911820733, 19.81200274180636711 ) ) ;
#14107=EDGE_CURVE ( 'NONE', #20820, #17548, #3132, .T. ) ;
#14126=CARTESIAN_POINT ( 'NONE',  ( 199.9999999999999716, 17.43237942262683049, 7.572151140094372401 ) ) ;
#14132=CARTESIAN_POINT ( 'NONE',  ( 199.0102239786929488, -4.226749394367478097, -19.54603893341629473 ) ) ;
#14140=CARTESIAN_POINT ( 'NONE',  ( 199.0223319294094892, 2.599958516019920118, 19.83413122362564351 ) ) ;
#14164=CARTESIAN_POINT ( 'NONE',  ( 199.9999999999998579, 18.23094931701148269, -5.355502299499542040 ) ) ;
#14165=CARTESIAN_POINT ( 'NONE',  ( 199.9999999999999432, -18.58351610408307764, -4.007049993893891049 ) ) ;
#14168=DIRECTION ( 'NONE',  ( -1.000000000000000000, -1.836970198721030181E-16, -2.465190328815661892E-32 ) ) ;
#14174=CARTESIAN_POINT ( 'NONE',  ( 199.0199791362716439, 7.640007438824279795, 18.48538610549022465 ) ) ;
#14175=CARTESIAN_POINT ( 'NONE',  ( -56.48582580120559271, 21.81201906317798489, -21.81201906317746619 ) ) ;
#14177=CARTESIAN_POINT ( 'NONE',  ( -192.9588430854690273, 66.79921049724377724, -10.23066800231904239 ) ) ;
#14189=CARTESIAN_POINT ( 'NONE',  ( 200.0000000000005400, -16.47398309245309278, 9.506867245997410620 ) ) ;
#14194=CARTESIAN_POINT ( 'NONE',  ( 199.0087111817176435, -0.6649071253763039202, -19.99597453042600392 ) ) ;
#14221=CARTESIAN_POINT ( 'NONE',  ( 199.9999999999997442, 15.07190321012488887, 11.58049570127731798 ) ) ;
#14227=CARTESIAN_POINT ( 'NONE',  ( 4.995406935893297984, 10.78321810390233892, -67.35176059882522281 ) ) ;
#14228=CARTESIAN_POINT ( 'NONE',  ( 199.0263607205240532, -13.20175300279655062, 15.04466839055514527 ) ) ;
#14255=CARTESIAN_POINT ( 'NONE',  ( 199.9999999999999432, 15.44072620018067887, 11.08370022558889545 ) ) ;
#14261=CARTESIAN_POINT ( 'NONE',  ( 199.0070327355206246, 4.219744681889460836, -19.54794762927634366 ) ) ;
#14271=CARTESIAN_POINT ( 'NONE',  ( 199.0156213727907186, 14.58859942632390094, 13.68185500382998576 ) ) ;
#14299=CARTESIAN_POINT ( 'NONE',  ( 199.9999999999998010, 13.53697630789494255, 13.34066885590318030 ) ) ;
#14300=CARTESIAN_POINT ( 'NONE',  ( 199.9999999999998863, -9.911147489498389973, -16.22017844385999297 ) ) ;
#14309=CARTESIAN_POINT ( 'NONE',  ( 199.0176277365346778, 11.71792290964084060, 16.22639131207622754 ) ) ;
#14310=CARTESIAN_POINT ( 'NONE',  ( -30.26275506840325136, 57.76657404653985139, -1.198031551615314161 ) ) ;
#14312=CARTESIAN_POINT ( 'NONE',  ( -135.8532207217289738, 21.81201906317729566, 34.75652343174635917 ) ) ;
#14327=CARTESIAN_POINT ( 'NONE',  ( 199.0168191192024949, -15.25344411108907572, -12.94054329384263724 ) ) ;
#14357=CARTESIAN_POINT ( 'NONE',  ( 200.0000000000003695, 4.006257452897062699, 18.58368358710308144 ) ) ;
#14363=CARTESIAN_POINT ( 'NONE',  ( 14.38125909742181285, -17.55144818341421598, -39.01709431150935359 ) ) ;
#14364=CARTESIAN_POINT ( 'NONE',  ( 199.0263115711520072, -12.44642065545630238, 15.66510279686564289 ) ) ;
#14387=( NAMED_UNIT ( * ) PLANE_ANGLE_UNIT ( ) SI_UNIT ( $, .RADIAN. ) );
#14389=EDGE_LOOP ( 'NONE', ( #23301, #7306 ) ) ;
#14390=CARTESIAN_POINT ( 'NONE',  ( 199.9999999999999716, 7.398602371178625958, 17.50881939353996231 ) ) ;
#14396=CARTESIAN_POINT ( 'NONE',  ( 199.0130599948309680, -9.716555752287060699, -17.48250520384952367 ) ) ;
#14406=CARTESIAN_POINT ( 'NONE',  ( 199.0221265002223845, 3.088699012602908578, 19.76381171561452632 ) ) ;
#14431=CARTESIAN_POINT ( 'NONE',  ( 199.9999999999997442, 17.78964944107278967, -6.681507572083275726 ) ) ;
#14433=CARTESIAN_POINT ( 'NONE',  ( 199.9999999999999716, 2.628281398024471027, -18.82296940602922675 ) ) ;
#14443=CARTESIAN_POINT ( 'NONE',  ( 199.0199344320482453, 7.725485862940699278, 18.44984083464702351 ) ) ;
#14446=CARTESIAN_POINT ( 'NONE',  ( -280.0000000000000000, 14.14213562373108246, -14.14213562373078581 ) ) ;
#14448=CARTESIAN_POINT ( 'NONE',  ( 163.1118516004056573, 37.29075403953132906, 19.27778845539275565 ) ) ;
#14460=CARTESIAN_POINT ( 'NONE',  ( 199.0082207658673781, 0.6402583678929150146, -19.98857080023024579 ) ) ;
#14486=CARTESIAN_POINT ( 'NONE',  ( 199.9999999999996874, 18.57765777299087873, -3.990914148134230288 ) ) ;
#14491=CARTESIAN_POINT ( 'NONE',  ( 146.6084372240433993, -24.48358557860353457, 24.48358557860296258 ) ) ;
#14492=CARTESIAN_POINT ( 'NONE',  ( 199.0249982833957176, -5.192600369583379560, 19.31944532238548362 ) ) ;
#14505=CARTESIAN_POINT ( 'NONE',  ( 199.0262120803540995, -11.39568569719682145, 16.44280778893389439 ) ) ;
#14518=CARTESIAN_POINT ( 'NONE',  ( 199.9999999999999147, -5.232840745185569631, 18.27603213255494552 ) ) ;
#14525=CARTESIAN_POINT ( 'NONE',  ( 199.0168191192024949, -15.25344411108907572, -12.94054329384263724 ) ) ;
#14538=CARTESIAN_POINT ( 'NONE',  ( 199.0070875033960078, 19.58406838943379569, -4.039067077891903779 ) ) ;
#14551=CARTESIAN_POINT ( 'NONE',  ( 199.0132069300353805, -9.958817830381372360, -17.35495257061628038 ) ) ;
#14561=CARTESIAN_POINT ( 'NONE',  ( 199.9999999999998863, -3.863658434880562265, -18.60611098383053630 ) ) ;
#14562=CARTESIAN_POINT ( 'NONE',  ( 199.9999999999998863, 13.43021917686961331, -13.43983678748323918 ) ) ;
#14571=CARTESIAN_POINT ( 'NONE',  ( 199.0084504823431359, 19.99625238461678478, -0.02475617773853401246 ) ) ;
#14573=CARTESIAN_POINT ( 'NONE',  ( 57.59792236341147031, 26.56190807104720975, -26.56190807104655249 ) ) ;
#14575=CARTESIAN_POINT ( 'NONE',  ( -56.48582580120559982, 50.09629031063956717, 6.472252184284792875 ) ) ;
#14588=CARTESIAN_POINT ( 'NONE',  ( 199.0260304748864257, -17.33599623264176870, 10.00424117181305128 ) ) ;
#14613=CARTESIAN_POINT ( 'NONE',  ( 200.0000000000000853, 16.14603016630555743, -10.01676266068942667 ) ) ;
#14618=CARTESIAN_POINT ( 'NONE',  ( 199.0254609980498799, -7.058152949095585882, 18.72097443096651403 ) ) ;
#14630=CARTESIAN_POINT ( 'NONE',  ( 199.0260264921024316, -10.00558763687667962, 17.32375098348098419 ) ) ;
#14643=CARTESIAN_POINT ( 'NONE',  ( 200.0000000000000284, 4.005278531425509492, 18.58194003000864569 ) ) ;
#14649=CARTESIAN_POINT ( 'NONE',  ( 199.0260304748864257, -17.33599623264176870, 10.00424117181305128 ) ) ;
#14656=AXIS2_PLACEMENT_3D ( 'NONE', #20675, #4448, #8420 ) ;
#14659=DIRECTION ( 'NONE',  ( -1.000000000000000000, -1.836970198721030181E-16, -2.465190328815661892E-32 ) ) ;
#14660=CARTESIAN_POINT ( 'NONE',  ( 199.0065089264240044, 19.04284699271596537, -6.106433644136123995 ) ) ;
#14668=AXIS2_PLACEMENT_3D ( 'NONE', #19880, #3393, #9903 ) ;
#14680=CARTESIAN_POINT ( 'NONE',  ( 199.0119150821959124, -7.654620711488286489, -18.47502128564530466 ) ) ;
#14694=CARTESIAN_POINT ( 'NONE',  ( 199.9999999999997726, 13.87428525677396607, -12.99608892921076198 ) ) ;
#14696=CARTESIAN_POINT ( 'NONE',  ( 200.0000000000000000, 12.98760816711885724, -13.88210512389335527 ) ) ;
#14706=CARTESIAN_POINT ( 'NONE',  ( 199.0056809825925370, 17.31175780291549415, -10.02710580630489900 ) ) ;
#14707=CARTESIAN_POINT ( 'NONE',  ( 192.4448373802101173, -14.14213562375826605, -42.42640687116518450 ) ) ;
#14721=CARTESIAN_POINT ( 'NONE',  ( 199.0208257245452899, -19.09599194444923143, -5.955353076589812389 ) ) ;
#14748=CARTESIAN_POINT ( 'NONE',  ( 200.0000000000000853, 11.56430744387933274, -15.08818561847743922 ) ) ;
#14751=CARTESIAN_POINT ( 'NONE',  ( 151.7948205124836250, -23.49921654116371883, 23.49921654116317526 ) ) ;
#14752=CARTESIAN_POINT ( 'NONE',  ( 199.0156213727907186, 14.58859942632390094, 13.68185500382998576 ) ) ;
#14787=CARTESIAN_POINT ( 'NONE',  ( 199.0188446093723371, -17.48804260178791736, -9.712431339257729945 ) ) ;
#14798=CARTESIAN_POINT ( 'NONE',  ( 199.0128224874292471, 17.70345943908711561, 9.303337553156843853 ) ) ;
#14812=CARTESIAN_POINT ( 'NONE',  ( 199.0084563976654977, 0.009091564791348882152, -19.99625984770770160 ) ) ;
#14823=CARTESIAN_POINT ( 'NONE',  ( 199.9999999999998863, 12.98615309696526587, -13.88358464575571283 ) ) ;
#14834=CARTESIAN_POINT ( 'NONE',  ( 199.0142575219002765, 16.25768778350697374, 11.67280966210075910 ) ) ;
#14835=CARTESIAN_POINT ( 'NONE',  ( -105.3755690713226727, -15.38646221621807619, 15.38646221621768362 ) ) ;
#14851=CARTESIAN_POINT ( 'NONE',  ( 199.0263554293247523, -15.04073044714995611, 13.19117051905602089 ) ) ;
#14868=FACE_OUTER_BOUND ( 'NONE', #2280, .T. ) ;
#14880=CARTESIAN_POINT ( 'NONE',  ( 199.9999999999997726, 7.546454185142647653, -17.43816512261951956 ) ) ;
#14883=CARTESIAN_POINT ( 'NONE',  ( 170.2234770963711128, -17.36149277827010096, 17.36149277826970660 ) ) ;
#14884=CARTESIAN_POINT ( 'NONE',  ( 199.0193391886810446, 8.833261569310058903, 17.94623560139499574 ) ) ;
#14910=CARTESIAN_POINT ( 'NONE',  ( 200.0000000000000000, -11.58160531504706547, 15.07837909557420275 ) ) ;
#14916=CARTESIAN_POINT ( 'NONE',  ( 199.0230409161751197, -19.98726064469808961, -0.8218112272605428981 ) ) ;
#14932=CARTESIAN_POINT ( 'NONE',  ( 199.0120816426991155, 18.34336195414084969, 7.966874786652939910 ) ) ;
#14961=CARTESIAN_POINT ( 'NONE',  ( 200.0000000000002842, 4.912815075579886503, -18.35721014059308942 ) ) ;
#14962=CARTESIAN_POINT ( 'NONE',  ( 199.9999999999999147, -4.322471944100380270, -18.50700405022334394 ) ) ;
#14970=CARTESIAN_POINT ( 'NONE',  ( 199.0084341825046579, 19.99614386575786895, -0.06800903924364970488 ) ) ;
#14971=CARTESIAN_POINT ( 'NONE',  ( 14.38125909742180752, 10.73282306404735387, -10.73282306404708919 ) ) ;
#14985=CARTESIAN_POINT ( 'NONE',  ( 199.0263429660336385, -15.25543418246514982, 12.94225785457335753 ) ) ;
#15015=CARTESIAN_POINT ( 'NONE',  ( 199.9999999999998579, 18.35745069958362308, -4.904641354906189576 ) ) ;
#15019=CARTESIAN_POINT ( 'NONE',  ( 199.0166590359707754, 13.17187519532568984, 15.05399639075651130 ) ) ;
#15034=CARTESIAN_POINT ( 'NONE',  ( -198.0356074513804572, 39.15871834505887250, 17.40982414986519089 ) ) ;
#15045=CARTESIAN_POINT ( 'NONE',  ( 199.9999999999999716, 1.537950039062797591, 18.94885247980957743 ) ) ;
#15051=CARTESIAN_POINT ( 'NONE',  ( 199.0231033154536817, -19.99336494683761956, -0.6578043788800663760 ) ) ;
#15062=CARTESIAN_POINT ( 'NONE',  ( 199.0054082256929746, 12.16974446990029790, -15.87805152391047159 ) ) ;
#15077=CARTESIAN_POINT ( 'NONE',  ( 199.0114802890556120, -6.820031933092490561, -18.79972423194800513 ) ) ;
#15087=CARTESIAN_POINT ( 'NONE',  ( 199.9999999999999147, -4.475453068641236598, -18.46865746885900705 ) ) ;
#15097=CARTESIAN_POINT ( 'NONE',  ( 199.0119184457754500, 18.47239636957207409, 7.660959720935172967 ) ) ;
#15098=CARTESIAN_POINT ( 'NONE',  ( 163.1118516004056573, -19.27778845539181063, -37.29075403953176959 ) ) ;
#15115=CARTESIAN_POINT ( 'NONE',  ( 200.0000000000000000, 12.97704027674654270, 13.88623514161034045 ) ) ;
#15117=CARTESIAN_POINT ( 'NONE',  ( 199.9999999999999147, -11.82758851212937579, 14.88619241608240529 ) ) ;
#15143=CARTESIAN_POINT ( 'NONE',  ( 199.9999999999999716, -9.233471789954972309, -16.61280101608961246 ) ) ;
#15147=CARTESIAN_POINT ( 'NONE',  ( 199.0099419815959436, 19.67222971740176618, 3.604179563970075773 ) ) ;
#15165=CARTESIAN_POINT ( 'NONE',  ( 199.0251223662492635, -5.665586242881555101, 19.18612710904600149 ) ) ;
#15167=CARTESIAN_POINT ( 'NONE',  ( 57.59792236341147031, -1.722363176415055985, 1.722363176415024677 ) ) ;
#15173=( NAMED_UNIT ( * ) PLANE_ANGLE_UNIT ( ) SI_UNIT ( $, .RADIAN. ) );
#15183=CARTESIAN_POINT ( 'NONE',  ( 199.9999999999996021, 1.536416165433052594, 18.94899354046687279 ) ) ;
#15211=CARTESIAN_POINT ( 'NONE',  ( 199.0176169432867255, -16.21418787309026754, -11.73480061161339272 ) ) ;
#15219=CARTESIAN_POINT ( 'NONE',  ( 200.0000000000001990, -15.45587892757197146, -11.06220582312848144 ) ) ;
#15228=CARTESIAN_POINT ( 'NONE',  ( 200.0000000000000000, -14.14213562373046784, -42.42640687119298804 ) ) ;
#15243=CARTESIAN_POINT ( 'NONE',  ( 199.9999999999998863, -2.178116022715518074, 18.88665387132288487 ) ) ;
#15270=CARTESIAN_POINT ( 'NONE',  ( 200.0000000000002558, -1.250172057809772586, -18.97074946354465652 ) ) ;
#15274=CARTESIAN_POINT ( 'NONE',  ( 199.0056246187962188, 17.07746298573517052, -10.40099104823843312 ) ) ;
#15288=CARTESIAN_POINT ( 'NONE',  ( 4.995406935893289102, 10.78321810389013002, -10.78321810388986712 ) ) ;
#15294=MECHANICAL_DESIGN_GEOMETRIC_PRESENTATION_REPRESENTATION('',(#442),#12327);
#15303=CARTESIAN_POINT ( 'NONE',  ( 199.9999999999998579, -4.480715147297966716, 18.47471730767352938 ) ) ;
#15305=ADVANCED_FACE ( 'NONE', ( #17766 ), #23369, .F. ) ;
#15334=CARTESIAN_POINT ( 'NONE',  ( 199.0179802867041019, -16.61558597860446440, -11.15304595324047554 ) ) ;
#15345=CARTESIAN_POINT ( 'NONE',  ( -198.0356074513804572, 39.15871834505956173, -39.15871834505865223 ) ) ;
#15347=CARTESIAN_POINT ( 'NONE',  ( 199.9999999999997442, -19.00693066143141152, -0.3125757794583984839 ) ) ;
#15373=CARTESIAN_POINT ( 'NONE',  ( 199.9999999999998010, 4.909892096549036467, 18.36538930945351566 ) ) ;
#15397=CARTESIAN_POINT ( 'NONE',  ( 199.9999999999997442, 1.230017881244859446, -18.96210773722240361 ) ) ;
#15400=CARTESIAN_POINT ( 'NONE',  ( 199.0055651108938832, 16.81514173603054374, -10.81990435933588302 ) ) ;
#15426=CARTESIAN_POINT ( 'NONE',  ( 200.0000000000000000, 2.003163845861910097, 18.90332168644373567 ) ) ;
#15433=DIRECTION ( 'NONE',  ( 0.000000000000000000, -1.000000000000000000, 0.000000000000000000 ) ) ;
#15463=CARTESIAN_POINT ( 'NONE',  ( 184.5686700507837656, 13.43430831934472103, -13.43430831934435510 ) ) ;
#15465=CARTESIAN_POINT ( 'NONE',  ( 200.0000000000000568, -11.58056098922197563, -15.07187815445410806 ) ) ;
#15490=CARTESIAN_POINT ( 'NONE',  ( 200.0000000000000000, 9.224923989862913842, 16.61864493261536424 ) ) ;
#15515=CARTESIAN_POINT ( 'NONE',  ( 200.0000000000001421, -12.54320094651582451, -14.29122475987005458 ) ) ;
#15518=CARTESIAN_POINT ( 'NONE',  ( 199.0058386706367912, 17.79887573832666092, -9.116163937183429766 ) ) ;
#15539=CARTESIAN_POINT ( 'NONE',  ( -238.4067589809705794, 0.6820004457912851592, -0.6820004457913123597 ) ) ;
#15550=CARTESIAN_POINT ( 'NONE',  ( 199.9999999999998010, -4.783743133932452096, 18.39862578376663294 ) ) ;
#15583=CARTESIAN_POINT ( 'NONE',  ( 199.0212986000439059, -19.41582075653976958, -4.984890382579185264 ) ) ;
#15590=CARTESIAN_POINT ( 'NONE',  ( -259.2033419157646676, 21.55415060305860209, -21.55415060305812602 ) ) ;
#15592=CARTESIAN_POINT ( 'NONE',  ( 199.9999999999998295, -7.847915761074617080, -17.31000481134407565 ) ) ;
#15604=CARTESIAN_POINT ( 'NONE',  ( 151.7948205124836250, -23.49921654116371883, 23.49921654116317526 ) ) ;
#15619=CARTESIAN_POINT ( 'NONE',  ( 199.9999999999998010, -4.783743133932452096, 18.39862578376663294 ) ) ;
#15633=CARTESIAN_POINT ( 'NONE',  ( 184.8905102610680444, -14.79361573936399665, 14.79361573936367158 ) ) ;
#15643=CARTESIAN_POINT ( 'NONE',  ( 200.0000000000001137, -7.564955314186367907, -17.43543124971759539 ) ) ;
#15646=EDGE_CURVE ( 'NONE', #15869, #8765, #11456, .T. ) ;
#15649=CARTESIAN_POINT ( 'NONE',  ( 199.0053213077726753, 13.66600449016087993, -14.61040478752057226 ) ) ;
#15678=CARTESIAN_POINT ( 'NONE',  ( 200.0000000000000568, -10.82911035642265141, 15.62521814345774196 ) ) ;
#15708=CARTESIAN_POINT ( 'NONE',  ( 200.0000000000000000, 15.11283142964146364, -11.58284877839162519 ) ) ;
#15709=CARTESIAN_POINT ( 'NONE',  ( 199.0254332542744464, -18.76228886362404324, 6.941650229743832057 ) ) ;
#15719=CARTESIAN_POINT ( 'NONE',  ( -30.26275506840323715, 29.48230279907829754, -29.48230279907758344 ) ) ;
#15748=CARTESIAN_POINT ( 'NONE',  ( 199.9999999999996874, -6.995992324030534171, 17.67857064404661926 ) ) ;
#15760=CARTESIAN_POINT ( 'NONE',  ( -135.8532207217289738, 50.09629031063956006, 6.472252184284782217 ) ) ;
#15763=CARTESIAN_POINT ( 'NONE',  ( -86.96347745069644475, -15.38646221621807442, 15.38646221621768184 ) ) ;
#15773=CARTESIAN_POINT ( 'NONE',  ( 199.9999999999999432, -13.87586802671829211, 12.99819774096606118 ) ) ;
#15776=CARTESIAN_POINT ( 'NONE',  ( 199.0067595892537327, 5.170136663293450674, -19.31817980730454209 ) ) ;
#15798=CARTESIAN_POINT ( 'NONE',  ( 170.2234770963711128, -17.36149277827010096, 17.36149277826970660 ) ) ;
#15808=CARTESIAN_POINT ( 'NONE',  ( 200.0000000000000000, 17.99290950227088004, 6.120759354987654000 ) ) ;
#15814=CARTESIAN_POINT ( 'NONE',  ( 14.38125909742181463, 10.73282306403652875, -67.30136555895941797 ) ) ;
#15851=CARTESIAN_POINT ( 'NONE',  ( 199.0207542291320522, 6.104323864361830942, 19.05092312409432154 ) ) ;
#15869=VERTEX_POINT ( 'NONE', #1806 ) ;
#15881=CARTESIAN_POINT ( 'NONE',  ( 199.9999999999998579, 17.43084440603007224, 7.570815656493459223 ) ) ;
#15883=CARTESIAN_POINT ( 'NONE',  ( 199.9999999999999147, -16.15527612753063380, 10.03904652186156099 ) ) ;
#15893=CARTESIAN_POINT ( 'NONE',  ( 199.0255668866977032, -7.539808606132146096, 18.52949269774865471 ) ) ;
#15895=CARTESIAN_POINT ( 'NONE',  ( -100.7734535825088500, 12.25131212657428748, 44.31723036834913643 ) ) ;
#15907=CARTESIAN_POINT ( 'NONE',  ( 200.0000000000001137, -18.99355687379454949, 0.7833857536329088544 ) ) ;
#15911=CARTESIAN_POINT ( 'NONE',  ( 199.0161314855084527, -14.37392100214799839, -13.91043101682956973 ) ) ;
#15940=CARTESIAN_POINT ( 'NONE',  ( 200.0000000000000000, 15.44098642598172866, 11.08330662512073950 ) ) ;
#15945=ADVANCED_FACE ( 'NONE', ( #1671 ), #17880, .F. ) ;
#15949=CARTESIAN_POINT ( 'NONE',  ( 199.9999999999999432, 14.14213562373110911, -14.14213562373072364 ) ) ;
#15977=DIRECTION ( 'NONE',  ( 1.000000000000000000, 0.000000000000000000, 0.000000000000000000 ) ) ;
#15980=CARTESIAN_POINT ( 'NONE',  ( 199.9999999999999147, 17.78310516339310254, 6.706406138798904237 ) ) ;
#15987=CARTESIAN_POINT ( 'NONE',  ( 199.0067595892537327, 5.170136663293450674, -19.31817980730454209 ) ) ;
#15992=DIRECTION ( 'NONE',  ( 0.000000000000000000, -0.7071067811865561215, 0.7071067811865389130 ) ) ;
#15994=CARTESIAN_POINT ( 'NONE',  ( 200.0000000000001137, -18.36608873747554327, 4.914565663504686377 ) ) ;
#15998=CARTESIAN_POINT ( 'NONE',  ( 199.0245441510845410, -3.586860678693493565, 19.68275873856094549 ) ) ;
#16024=CARTESIAN_POINT ( 'NONE',  ( 200.0000000000000000, 17.99825158093497635, -6.097534595090909448 ) ) ;
#16025=CARTESIAN_POINT ( 'NONE',  ( 199.9999999999999432, -17.05147999913141277, 8.410089918960904853 ) ) ;
#16034=CARTESIAN_POINT ( 'NONE',  ( 199.0186595897608868, 10.02499462136977115, 17.31996783451393540 ) ) ;
#16035=CARTESIAN_POINT ( 'NONE',  ( -30.26275506840324070, 1.198031551616724366, -57.76657404653984429 ) ) ;
#16038=CARTESIAN_POINT ( 'NONE',  ( 91.82158438592158234, -12.16597498397778843, 12.16597498397750954 ) ) ;
#16049=CARTESIAN_POINT ( 'NONE',  ( 200.0000000000002558, -14.49689853580991539, 12.29876589910006857 ) ) ;
#16054=CARTESIAN_POINT ( 'NONE',  ( 199.0101504891794946, -4.065683697617192394, -19.58013257009994135 ) ) ;
#16082=CARTESIAN_POINT ( 'NONE',  ( 199.9999999999998295, 10.02997355460652429, 16.14748021227288532 ) ) ;
#16088=CARTESIAN_POINT ( 'NONE',  ( 136.1360204305621551, -24.77266263493081766, -31.79587985999290112 ) ) ;
#16089=CARTESIAN_POINT ( 'NONE',  ( 199.0227319893622848, 1.617020328492027259, 19.94056979940310015 ) ) ;
#16115=CARTESIAN_POINT ( 'NONE',  ( 199.9999999999999147, 18.88155072364786591, -2.150913467935055223 ) ) ;
#16121=CARTESIAN_POINT ( 'NONE',  ( 199.0100048860339541, -3.743224330709818748, -19.64425440907078269 ) ) ;
#16127=CARTESIAN_POINT ( 'NONE',  ( 200.0000000000003411, -18.28334586770733594, 5.214203034309022655 ) ) ;
#16130=CARTESIAN_POINT ( 'NONE',  ( 199.0232347278000873, 0.3099713519423794028, 20.00382596759649800 ) ) ;
#16159=CARTESIAN_POINT ( 'NONE',  ( 200.0000000000002842, 18.39723030902092660, -4.753359243483134655 ) ) ;
#16160=CARTESIAN_POINT ( 'NONE',  ( 199.9999999999999432, -14.49604467618470593, -12.29544462711038832 ) ) ;
#16170=CARTESIAN_POINT ( 'NONE',  ( 199.0250287384835985, -5.300309701115731187, 19.29992413559400788 ) ) ;
#16171=CARTESIAN_POINT ( 'NONE',  ( 91.82158438592158234, 16.11829626346161604, -16.11829626346121103 ) ) ;
#16173=CARTESIAN_POINT ( 'NONE',  ( -208.1127848780264742, 67.17687982763172272, -10.60833733270698254 ) ) ;
#16186=CARTESIAN_POINT ( 'NONE',  ( 200.0000000000000284, -17.94985894478863386, -6.254032569489808679 ) ) ;
#16189=CARTESIAN_POINT ( 'NONE',  ( 199.0103724725597658, -4.548822225537863417, -19.47368150598642345 ) ) ;
#16207=B_SPLINE_CURVE_WITH_KNOTS ( 'NONE', 3,
 ( #2986, #2729, #10834, #18950, #24952, #731, #595, #6699, #8566, #16680, #8836, #25079, #16944, #4456, #6830, #4591, #6433, #23208, #13095, #24811, #12550, #19208, #12960, #21079, #20682, #10971, #14812, #19080, #860, #8969, #17078, #25212, #6960, #990, #15077, #22814, #4989, #21213, #2452, #2590, #18815, #6563, #14680, #11092, #16547, #12688, #24677, #14551, #22681, #10562, #18675, #461, #20818, #10705, #7468, #25853, #23834, #17710, #23707, #19847, #21587, #15211, #15334, #7097, #25596, #3358, #23582, #9348, #13339, #1500, #23338, #23463, #5114, #7343, #13219, #5234, #21340, #15583, #5616, #7597, #11589, #17202, #3111, #9095, #25340, #1243, #5359, #11340, #11216, #11460, #19330, #13722, #17456, #17580, #7218, #3618, #15709, #9224, #21847, #3235, #25716, #21460, #11729, #13466, #21714, #5486, #9473, #19711 ),
 .UNSPECIFIED., .F., .F.,
 ( 4, 2, 2, 2, 1, 1, 1, 2, 2, 2, 2, 2, 1, 1, 1, 1, 2, 2, 2, 2, 2, 1, 1, 1, 1, 1, 1, 2, 2, 2, 2, 2, 2, 2, 1, 2, 2, 2, 2, 2, 2, 1, 1, 1, 1, 1, 2, 2, 2, 2, 2, 1, 1, 1, 1, 2, 2, 2, 2, 2, 1, 1, 1, 2, 2, 2, 4 ),
 ( 0.5000000000000000000, 0.5312500000000124345, 0.5468750000000187628, 0.5546875000000218714, 0.5585937500000235367, 0.5605468750000243139, 0.5615234375000246470, 0.5620117187500248690, 0.5625000000000250910, 0.5937500000000373035, 0.6093750000000434097, 0.6171875000000464073, 0.6210937500000479616, 0.6230468750000487388, 0.6240234375000490719, 0.6245117187500492939, 0.6247558593750494049, 0.6250000000000495159, 0.6562500000000617284, 0.6718750000000678346, 0.6796875000000708322, 0.6835937500000723865, 0.6855468750000731637, 0.6865234375000734968, 0.6870117187500737188, 0.6872558593750738298, 0.6873779296875738298, 0.6874389648438239409, 0.6875000000000739409, 0.7031250000000741629, 0.7187500000000744960, 0.7343750000000748290, 0.7421875000000749401, 0.7460937500000750511, 0.7480468750000750511, 0.7490234375000750511, 0.7500000000000750511, 0.7656250000000757172, 0.7812500000000763833, 0.7968750000000770495, 0.8046875000000772715, 0.8085937500000774936, 0.8105468750000776046, 0.8115234375000776046, 0.8120117187500776046, 0.8122558593750776046, 0.8123779296875774936, 0.8125000000000774936, 0.8437500000000639488, 0.8593750000000570655, 0.8671875000000537348, 0.8710937500000519584, 0.8730468750000510703, 0.8740234375000506262, 0.8745117187500504041, 0.8747558593750504041, 0.8750000000000501821, 0.9062500000000366374, 0.9218750000000297540, 0.9296875000000264233, 0.9335937500000248690, 0.9355468750000239808, 0.9365234375000235367, 0.9370117187500233147, 0.9375000000000230926, 0.9687500000000115463, 1.000000000000000000 ),
 .UNSPECIFIED. ) ;
#16218=CARTESIAN_POINT ( 'NONE',  ( 199.9999999999999432, 3.548988777896260771, 18.67457114543681485 ) ) ;
#16226=CARTESIAN_POINT ( 'NONE',  ( 200.0000000000000000, -14.14213562373046784, -42.42640687119298804 ) ) ;
#16252=CARTESIAN_POINT ( 'NONE',  ( 199.9999999999999716, 18.27648386272512226, -5.205167537210750872 ) ) ;
#16258=CARTESIAN_POINT ( 'NONE',  ( 199.0078145870362221, 1.786107411569149317, -19.91668635079984284 ) ) ;
#16263=CARTESIAN_POINT ( 'NONE',  ( 199.9999999999999432, -13.66164182518334691, 13.22314710892283074 ) ) ;
#16266=CARTESIAN_POINT ( 'NONE',  ( 199.0186810464772691, 9.993108295904475469, 17.32680936265314386 ) ) ;
#16287=EDGE_CURVE ( 'NONE', #19850, #5454, #24821, .T. ) ;
#16294=CARTESIAN_POINT ( 'NONE',  ( 199.9999999999998863, 14.88114354045644561, 11.82478185164094775 ) ) ;
#16297=CARTESIAN_POINT ( 'NONE',  ( 200.0000000000000000, -18.00239984878453825, 6.108539637176261472 ) ) ;
#16306=CARTESIAN_POINT ( 'NONE',  ( 199.0258546901197860, -8.886439070910094884, 17.97156912711873034 ) ) ;
#16307=CARTESIAN_POINT ( 'NONE',  ( 146.6084372240433993, 3.800685668858732935, -3.800685668858610367 ) ) ;
#16309=CARTESIAN_POINT ( 'NONE',  ( 4.995406935893286438, 67.35176059880245703, -10.78321810387767066 ) ) ;
#16319=CARTESIAN_POINT ( 'NONE',  ( 199.9999999999999147, -17.67734251759716457, -6.986728219496066927 ) ) ;
#16322=CARTESIAN_POINT ( 'NONE',  ( 199.0135655005340425, -10.56572504866429973, -16.98073106299600710 ) ) ;
#16349=CARTESIAN_POINT ( 'NONE',  ( 199.9999999999999716, 15.96353534131429797, 10.31599105002992545 ) ) ;
#16355=CARTESIAN_POINT ( 'NONE',  ( 19.06497207195981147, 38.31983398719673772, -38.31983398719579981 ) ) ;
#16356=CARTESIAN_POINT ( 'NONE',  ( 199.0218477376944577, 3.734929907270702287, 19.65178994764128717 ) ) ;
#16383=CARTESIAN_POINT ( 'NONE',  ( 199.9999999999999147, 7.829686725388152801, 17.32023057510092912 ) ) ;
#16391=CARTESIAN_POINT ( 'NONE',  ( 199.0106728332879698, -5.188592077825961546, -19.31531804097554073 ) ) ;
#16404=CARTESIAN_POINT ( 'NONE',  ( 199.0151032989660678, 15.24552994868030531, 12.94849756636627447 ) ) ;
#16431=CARTESIAN_POINT ( 'NONE',  ( 199.9999999999999432, 17.49244587396685091, 7.427265670988617785 ) ) ;
#16432=CARTESIAN_POINT ( 'NONE',  ( 199.9999999999998863, -15.08414020386666721, -11.56687813556520261 ) ) ;
#16444=CARTESIAN_POINT ( 'NONE',  ( -238.4067589809705794, 28.96627169325354956, -28.96627169325289231 ) ) ;
#16446=CARTESIAN_POINT ( 'NONE',  ( 146.6084372240433709, 32.08495691632030145, 24.48358557860365181 ) ) ;
#16460=CARTESIAN_POINT ( 'NONE',  ( 199.0175917791061977, -16.16856137136818816, -11.77441583767826039 ) ) ;
#16484=ORIENTED_EDGE ( 'NONE', *, *, #8406, .F. ) ;
#16488=CARTESIAN_POINT ( 'NONE',  ( 199.9999999999998863, 3.552885321105354599, -18.66644157592937248 ) ) ;
#16494=CARTESIAN_POINT ( 'NONE',  ( -30.26275506840324070, 1.198031551616030033, -1.198031551616006496 ) ) ;
#16524=CARTESIAN_POINT ( 'NONE',  ( 199.0111317961331281, -6.131174403448985011, -19.03732645848564431 ) ) ;
#16535=CARTESIAN_POINT ( 'NONE',  ( 199.0064300139308102, 18.94043123351016433, -6.416860702434988184 ) ) ;
#16547=CARTESIAN_POINT ( 'NONE',  ( 199.0121230032554251, -8.046372254322770701, -18.31269210357472943 ) ) ;
#16560=CARTESIAN_POINT ( 'NONE',  ( 199.9999999999997442, 1.230017881244859446, -18.96210773722240361 ) ) ;
#16561=CARTESIAN_POINT ( 'NONE',  ( 199.9999999999999147, 10.03116143388543868, -16.13932148327019078 ) ) ;
#16570=CARTESIAN_POINT ( 'NONE',  ( 199.0116138701751538, 18.70391647836493476, 7.080528309964213562 ) ) ;
#16572=CARTESIAN_POINT ( 'NONE',  ( 136.1360204305621551, 31.79587985999232558, 24.77266263493161702 ) ) ;
#16574=CARTESIAN_POINT ( 'NONE',  ( 184.8905102610680444, 13.49065550809757497, 43.07788698682593065 ) ) ;
#16587=CARTESIAN_POINT ( 'NONE',  ( 199.0231033154536817, -19.99336494683761956, -0.6578043788800663760 ) ) ;
#16614=CARTESIAN_POINT ( 'NONE',  ( 200.0000000000002558, 17.05253901346626222, -8.385556056821480198 ) ) ;
#16620=CARTESIAN_POINT ( 'NONE',  ( -238.4067589809705794, -27.60227080167029001, -28.96627169325357798 ) ) ;
#16621=FACE_OUTER_BOUND ( 'NONE', #22020, .T. ) ;
#16637=CARTESIAN_POINT ( 'NONE',  ( 199.0261090282319856, -10.57113834583376644, 16.98461103275367634 ) ) ;
#16656=CARTESIAN_POINT ( 'NONE',  ( 199.0244488197511998, -19.74721217248383809, 3.261676333419620821 ) ) ;
#16667=CARTESIAN_POINT ( 'NONE',  ( 199.0072342795740497, 19.67962538453564036, -3.556093180948044274 ) ) ;
#16680=CARTESIAN_POINT ( 'NONE',  ( 199.0060826632022781, 7.907239936230238797, -18.36546223987650706 ) ) ;
#16690=CARTESIAN_POINT ( 'NONE',  ( 200.0000000000001990, 0.6082288760829889229, -18.99424756986708474 ) ) ;
#16691=CARTESIAN_POINT ( 'NONE',  ( 199.9999999999999716, -4.015339075642541111, -18.57593938989771587 ) ) ;
#16701=CARTESIAN_POINT ( 'NONE',  ( 199.0079644305843090, 19.95293258044705098, -1.355764268682818408 ) ) ;
#16702=CARTESIAN_POINT ( 'NONE',  ( -192.9588430854690273, -18.05360324515400094, -38.51493924976961836 ) ) ;
#16704=CARTESIAN_POINT ( 'NONE',  ( 170.2234770963711128, 10.92277846919147066, 45.64576402573197811 ) ) ;
#16717=CARTESIAN_POINT ( 'NONE',  ( 199.9999999999995453, -10.04557064260861843, 16.14007440661455206 ) ) ;
#16745=CARTESIAN_POINT ( 'NONE',  ( 199.9999999999998579, 15.71915069317562264, -10.67410001769982308 ) ) ;
#16749=CARTESIAN_POINT ( 'NONE',  ( 19.06497207195980792, -18.24870850772710540, -38.31983398719647482 ) ) ;
#16750=CARTESIAN_POINT ( 'NONE',  ( 199.0160554649137907, 14.01242985958090692, 14.27167877623515757 ) ) ;
#16763=CARTESIAN_POINT ( 'NONE',  ( 199.0263771359574889, -13.68429728450633753, 14.60718570525551563 ) ) ;
#16784=CARTESIAN_POINT ( 'NONE',  ( 199.0147604500337764, -12.44374936594963899, -15.65999889774876941 ) ) ;
#16797=CARTESIAN_POINT ( 'NONE',  ( 199.0123267138131098, 18.14094429105657369, 8.417911433729377890 ) ) ;
#16815=ORIENTED_EDGE ( 'NONE', *, *, #19870, .F. ) ;
#16826=CARTESIAN_POINT ( 'NONE',  ( 199.9999999999998010, 6.097523047862603462, -17.99825575681430223 ) ) ;
#16828=CARTESIAN_POINT ( 'NONE',  ( 199.9999999999999716, -7.851927509958055218, -17.31649898218073957 ) ) ;
#16840=CARTESIAN_POINT ( 'NONE',  ( 199.0058351560425365, 17.78440418358302111, -9.144608015618983288 ) ) ;
#16841=CARTESIAN_POINT ( 'NONE',  ( -162.0762913951020892, 1.198031840385732849, -1.198031840385733515 ) ) ;
#16847=ORIENTED_EDGE ( 'NONE', *, *, #26231, .T. ) ;
#16857=CARTESIAN_POINT ( 'NONE',  ( 199.0263189878286028, -15.57072488730636017, 12.56115478513486217 ) ) ;
#16883=CARTESIAN_POINT ( 'NONE',  ( 199.9999999999999716, 14.88808753490056880, -11.80862348214050606 ) ) ;
#16887=CARTESIAN_POINT ( 'NONE',  ( 199.0151032989660678, 15.24552994868030531, 12.94849756636627447 ) ) ;
#16913=CARTESIAN_POINT ( 'NONE',  ( 199.9999999999999716, 2.469089442616056562, 18.84997742926038455 ) ) ;
#16919=CARTESIAN_POINT ( 'NONE',  ( 199.0175917791061977, -16.16856137136818816, -11.77441583767826039 ) ) ;
#16930=CARTESIAN_POINT ( 'NONE',  ( 199.0058386706367912, 17.79887573832666092, -9.116163937183429766 ) ) ;
#16944=CARTESIAN_POINT ( 'NONE',  ( 199.0061329731654496, 7.677669731782176932, -18.46232380042365051 ) ) ;
#16956=CARTESIAN_POINT ( 'NONE',  ( 199.9999999999996021, 4.009690090792337180, -18.57554820616829261 ) ) ;
#16958=CARTESIAN_POINT ( 'NONE',  ( 200.0000000000000000, 1.231416217928662515, -18.97163116072034938 ) ) ;
#16968=CARTESIAN_POINT ( 'NONE',  ( 199.0053212086165502, 15.02621665087036362, -13.25052931267129885 ) ) ;
#16969=CARTESIAN_POINT ( 'NONE',  ( -30.26275506840324070, 1.198031551616030033, -1.198031551616006496 ) ) ;
#16983=CARTESIAN_POINT ( 'NONE',  ( 199.0207495982873809, -19.04631292825652622, -6.112231798784620196 ) ) ;
#16999=DIRECTION ( 'NONE',  ( 1.836970198721030181E-16, -1.000000000000000000, 0.000000000000000000 ) ) ;
#17010=CARTESIAN_POINT ( 'NONE',  ( 199.9999999999998579, 7.403094706059546226, -17.49952075364730675 ) ) ;
#17014=CARTESIAN_POINT ( 'NONE',  ( 199.0202951899208017, 7.027923415129357032, 18.72965638665138144 ) ) ;
#17031=CARTESIAN_POINT ( 'NONE',  ( -100.7734535825088500, 40.53558337403654832, 16.03295912088756481 ) ) ;
#17043=CARTESIAN_POINT ( 'NONE',  ( 199.9999999999999432, -6.708851862405343702, 17.79758909344539219 ) ) ;
#17048=CARTESIAN_POINT ( 'NONE',  ( 199.0200497209392267, -18.54142962866078648, -7.504851164020625021 ) ) ;
#17063=CARTESIAN_POINT ( 'NONE',  ( 199.0053213077726753, 13.66600449016087993, -14.61040478752057226 ) ) ;
#17078=CARTESIAN_POINT ( 'NONE',  ( 199.0102713619699841, -4.331938195896105626, -19.53328621734312875 ) ) ;
#17088=CARTESIAN_POINT ( 'NONE',  ( 200.0000000000001705, 6.971423609723053971, -17.67803530771774589 ) ) ;
#17089=CARTESIAN_POINT ( 'NONE',  ( 199.9999999999999432, 8.677819433020733442, -16.90353765624616500 ) ) ;
#17097=CARTESIAN_POINT ( 'NONE',  ( 199.0102747309263975, 19.53166102356907885, 4.339329946343584155 ) ) ;
#17098=CARTESIAN_POINT ( 'NONE',  ( 136.1360204305621551, -24.77266263493081766, -31.79587985999290112 ) ) ;
#17104=EDGE_CURVE ( 'NONE', #19850, #5806, #6209, .T. ) ;
#17115=CARTESIAN_POINT ( 'NONE',  ( 199.0263771353516233, -14.14574067859894413, 14.14574067859863682 ) ) ;
#17139=CARTESIAN_POINT ( 'NONE',  ( 200.0000000000000284, -14.89093438834758842, -11.81132417993805639 ) ) ;
#17144=CARTESIAN_POINT ( 'NONE',  ( 199.0123267138131098, 18.14094429105657369, 8.417911433729377890 ) ) ;
#17157=CARTESIAN_POINT ( 'NONE',  ( 199.0249982833957176, -5.192600369583379560, 19.31944532238548362 ) ) ;
#17159=CARTESIAN_POINT ( 'NONE',  ( -259.2033419157646676, 49.83842185052017015, 6.730120644404137487 ) ) ;
#17175=CARTESIAN_POINT ( 'NONE',  ( 199.0205961407162931, -18.94296041394271768, -6.425165802706580997 ) ) ;
#17202=CARTESIAN_POINT ( 'NONE',  ( 199.0228991319552563, -19.97028783757971127, -1.189345221019080245 ) ) ;
#17212=CARTESIAN_POINT ( 'NONE',  ( 199.9999999999999147, -15.17855064416508526, -11.43956010876637563 ) ) ;
#17224=CARTESIAN_POINT ( 'NONE',  ( -259.2033419157646676, -35.01439189186523748, -21.55415060305881170 ) ) ;
#17241=CARTESIAN_POINT ( 'NONE',  ( 199.9999999999998295, 0.2943743412949595961, 19.00910698902408669 ) ) ;
#17268=CARTESIAN_POINT ( 'NONE',  ( 200.0000000000000000, -14.79283710360616944, -11.93388616463377438 ) ) ;
#17273=CARTESIAN_POINT ( 'NONE',  ( 199.0155347402294410, 14.70064717653387554, 13.56132639103557125 ) ) ;
#17289=CARTESIAN_POINT ( 'NONE',  ( 130.8568914410475372, -24.07718906447255947, 24.07718906447199458 ) ) ;
#17293=ORIENTED_EDGE ( 'NONE', *, *, #6153, .F. ) ;
#17297=CARTESIAN_POINT ( 'NONE',  ( -259.2033419157646676, -6.730120644403663199, 6.730120644403451813 ) ) ;
#17306=CARTESIAN_POINT ( 'NONE',  ( 199.9999999999999147, -8.688421465551046552, 16.91138275242808575 ) ) ;
#17307=CARTESIAN_POINT ( 'NONE',  ( -280.0000000000000000, -14.14213562373118371, 14.14213562373078936 ) ) ;
#17344=CARTESIAN_POINT ( 'NONE',  ( 199.9999999999999147, -13.00175152101318510, -13.87559618198639022 ) ) ;
#17368=CARTESIAN_POINT ( 'NONE',  ( 199.9999999999999147, -9.100092698529554269, 16.69133291234032868 ) ) ;
#17392=CARTESIAN_POINT ( 'NONE',  ( 200.0000000000000284, -8.407999580957739028, -17.04516676560209376 ) ) ;
#17396=CARTESIAN_POINT ( 'NONE',  ( 199.0062801237116332, 7.031410157601610145, -18.72090521856086198 ) ) ;
#17409=B_SPLINE_SURFACE_WITH_KNOTS ( 'NONE', 1, 3, ( 
 ( #4273, #10111, #14228, #14364, #8238, #4144, #12361, #2395, #11971, #24754, #6374, #26236, #18212, #12236, #20492, #8106, #8373, #2135, #10373, #6508, #264, #18483, #14618, #6120, #18354, #3869, #22228, #14492, #20619, #24620, #18621, #2005, #10507, #1874, #22625, #4400, #20095, #12494, #20360, #9977, #18085, #7970, #16089, #24219, #22367, #5990, #14099, #134, #4004, #12103, #16356, #24489, #20227, #24356, #6251, #21152, #2797, #17014, #13034, #10773, #5053, #2668, #14884, #535, #1055, #7158, #25151, #12630, #800, #6902, #7028, #21279, #2926, #18886, #15019, #8640, #4799, #664, #16750, #19021, #8773, #14752, #17273, #20757, #16887, #22753, #23149, #22883, #12764, #12900, #25018, #21015, #4661, #11035, #11157, #4921, #20889, #17144, #9039, #24882, #10909, #2527, #25278, #6638, #8904, #19145, #6772, #15147, #19272, #18752, #4532, #929, #23277, #10644, #13159, #3050, #9160, #25406, #23023, #25787, #13786, #17522, #21921, #1703, #21654, #5179, #11282, #17778, #3426, #13530, #17914, #5681, #23524, #25924, #23648, #5427, #15518, #3304, #11527, #15274, #19652, #15400, #1438, #7405, #9537, #17646, #9810, #7537, #19522, #1307, #23404, #15649, #7284, #5296, #23774, #9415, #5551, #13404, #13660, #3693, #21783, #21529, #9674, #1569, #9290, #3556, #13282, #7665, #17396, #11659, #19783, #25660, #15776, #11799, #19403, #21404, #23905, #19919, #3177, #26057, #1185, #25535, #11399, #8204, #18314, #6338, #10075, #14460, #20585, #14194, #24043, #3832, #10339, #22326, #6087, #10473, #24582, #16054, #18448, #16189, #24322, #8070, #22194, #4101, #7795, #12202, #7936, #20323, #26329, #2100, #10209, #2360, #96, #12068, #16322, #12458, #18180, #24449, #18588, #26199, #224, #22591, #6215, #4368, #5954, #15911, #5821, #8338, #14327, #13924, #20457, #22459, #22059, #16460, #11933, #2231, #20060, #4239, #1837, #9938, #12329, #18046, #24179, #14063, #3971, #20186, #1970, #22853, #25119, #6739, #20985, #16983, #14721, #9008, #6601, #18853, #4493, #5023, #11131, #2766, #16587, #4763, #10875, #11005, #25245, #6871, #4628, #18989, #12595, #8739, #12731, #20725, #22987, #20853, #18716, #21249, #24719, #2898, #6474, #13001, #8468, #10742, #6996, #14588, #12867, #23248, #365, #2633, #633, #4891, #16857, #24988, #14985, #14851, #767, #23119, #8873, #17115 ),
 ( #21121, #19115, #898, #15117, #8608, #13128, #10604, #22716, #3024, #2493, #501, #16717, #24849, #21885, #11499, #25761, #17368, #5270, #17491, #19625, #23374, #15748, #1410, #17616, #13373, #5150, #19370, #7254, #15619, #3662, #7633, #5652, #11372, #19244, #25379, #13255, #15243, #25633, #21378, #17241, #9646, #3148, #19751, #11251, #1027, #23742, #7379, #9126, #1541, #13501, #25892, #1157, #23876, #15373, #13758, #3399, #25505, #9261, #9511, #7131, #19493, #23496, #21503, #3274, #1277, #9384, #15490, #21623, #7509, #5523, #23618, #5400, #13630, #21754, #3528, #11629, #17749, #19889, #8305, #14299, #7767, #18016, #12038, #12175, #26164, #16294, #10047, #18284, #24557, #8179, #8042, #6060, #4209, #22433, #1807, #24420, #20029, #18152, #20295, #15881, #16431, #2073, #10180, #5926, #24008, #11904, #7905, #6184, #22561, #197, #6312, #3941, #11770, #17881, #5788, #13895, #26300, #22029, #9779, #2206, #3802, #12300, #9910, #1672, #20427, #16159, #26030, #10315, #14164, #18421, #16024, #14431, #24149, #14033, #22297, #22164, #20158, #70, #1939, #24293, #4073, #8579, #2464, #20560, #19092, #605, #24963, #18962, #22955, #10574, #14694, #14823, #8712, #4603, #4733, #2874, #12432, #872, #6841, #337, #18689, #12700, #12843, #473, #8847, #2602, #10844, #17088, #743, #16826, #6709, #23096, #14961, #20696, #16956, #12563, #10716, #8980, #2331, #10441, #8441, #22827, #18558, #25220, #4867, #16560, #6973, #16690, #20828, #20959, #24688, #2740, #24822, #6445, #12971, #25094, #6575, #14561, #21092, #10982, #15087, #18825, #4340, #22692, #4467, #9236, #17466, #3246, #15592, #25727, #11602, #5126, #5244, #7107, #11102, #7479, #9618, #21225, #1000, #19725, #25863, #15465, #3369, #21353, #17344, #21468, #9103, #19219, #11350, #25350, #2998, #13598, #17212, #23717, #15219, #4999, #1384, #19466, #13104, #5498, #25609, #3504, #23349, #1511, #19342, #17722, #7352, #3122, #13230, #13476, #11226, #23473, #7607, #1132, #25480, #7229, #23220, #1253, #23592, #11470, #5371, #15347, #13349, #21598, #9357, #19596, #9485, #21728, #17589, #12274, #18255, #11739, #21998, #15994, #16127, #3768, #20266, #14001, #22268, #2176, #12142, #12011, #10014, #8148, #36, #5757, #2045, #23980, #22131, #4180, #13732, #5626, #19858, #7872, #21858, #20402, #16263, #3632 ) ),
 .UNSPECIFIED., .F., .T., .F.,
 ( 2, 2 ),
 ( 4, 2, 2, 2, 2, 2, 2, 2, 2, 2, 2, 2, 2, 2, 2, 2, 2, 2, 2, 2, 2, 2, 2, 2, 2, 2, 2, 2, 2, 2, 2, 2, 2, 2, 2, 2, 2, 2, 2, 2, 2, 2, 2, 2, 2, 2, 2, 2, 2, 2, 2, 2, 2, 2, 2, 2, 2, 2, 2, 2, 2, 2, 2, 2, 2, 2, 2, 2, 2, 2, 2, 2, 2, 2, 2, 2, 2, 2, 2, 2, 2, 2, 2, 2, 2, 2, 2, 2, 2, 2, 2, 2, 2, 2, 2, 2, 2, 2, 2, 2, 2, 2, 2, 2, 2, 2, 2, 2, 2, 2, 2, 2, 2, 2, 2, 2, 2, 2, 2, 2, 2, 2, 2, 2, 2, 2, 2, 2, 2, 2, 2, 2, 2, 2, 2, 2, 2, 2, 2, 2, 2, 2, 2, 2, 2, 2, 2, 2, 4 ),
 ( 0.000000000000000000, 1.000000000000000000 ),
 ( 0.001986339241202381145, 0.003842975313193646575, 0.004771293349189279290, 0.005235452367187095647, 0.005699611385184912005, 0.006163770403182728362, 0.006627929421180544720, 0.007092088439178361077, 0.007556247457176177434, 0.008484565493171810149, 0.009412883529167442864, 0.01034120156516307558, 0.01126951960115870829, 0.01173367861915652552, 0.01219783763715434101, 0.01266199665515215650, 0.01312615567314997372, 0.01405447370914560644, 0.01498279174514123915, 0.01683942781713250458, 0.01776774585312813903, 0.01869606388912377001, 0.01916022290712158377, 0.01962438192511940099, 0.02008854094311721822, 0.02055269996111503544, 0.02148101799711066989, 0.02240933603310630087, 0.02333765406910193185, 0.02426597210509756630, 0.02519429014109320075, 0.02565844915909101798, 0.02612260817708883173, 0.02658676719508664549, 0.02705092621308446271, 0.02797924424908009716, 0.02983588032107136259, 0.03076419835706699357, 0.03122835737506481080, 0.03169251639306262802, 0.03215667541106044525, 0.03262083442905826247, 0.03354915246505389692, 0.03447747050104953137, 0.03540578853704515888, 0.03633410657304078639, 0.03726242460903642084, 0.03772658362703423807, 0.03819074264503205529, 0.03865490166302987252, 0.03911906068102768974, 0.04004737871702332419, 0.04097569675301895864, 0.04283233282501022060, 0.04376065086100584811, 0.04468896889700148256, 0.04561728693299711701, 0.04654560496899275146, 0.04840224104098402036, 0.04933055907697965481, 0.05025887711297528232, 0.05072303613097309261, 0.05118719514897090983, 0.05165135416696872706, 0.05211551318496654428, 0.05304383122096217873, 0.05397214925695781318, 0.05490046729295344763, 0.05582878532894908208, 0.05675710336494471653, 0.05722126238294253375, 0.05768542140094034404, 0.05814958041893815432, 0.05861373943693597155, 0.05954205747293160600, 0.06139869354492287490, 0.06325532961691412992, 0.06511196568890539882, 0.06604028372490103327, 0.06696860176089666772, 0.06743276077889448494, 0.06789691979689230217, 0.06836107881489011939, 0.06882523783288793662, 0.06975355586888357107, 0.07068187390487920552, 0.07161019194087483997, 0.07253850997687047442, 0.07300266899486829164, 0.07346682801286610887, 0.07393098703086392609, 0.07439514604886174332, 0.07485930506685956054, 0.07532346408485737776, 0.07625178212085299834, 0.07810841819284425336, 0.07903673622883988781, 0.07950089524683770503, 0.07996505426483552226, 0.08042921328283333948, 0.08089337230083115671, 0.08182169033682679116, 0.08275000837282242561, 0.08367832640881806006, 0.08460664444481369451, 0.08553496248080932896, 0.08646328051680496340, 0.08692743953480278063, 0.08739159855280059785, 0.08785575757079841508, 0.08831991658879623230, 0.08924823462479186675, 0.09110487069678312178, 0.09203318873277874235, 0.09296150676877437680, 0.09342566578677219402, 0.09388982480477001125, 0.09435398382276782847, 0.09481814284076564570, 0.09574646087676128015, 0.09667477891275691460, 0.09760309694875254904, 0.09853141498474818349, 0.09899557400274600072, 0.09945973302074381794, 0.09992389203874163517, 0.1003880510567394524, 0.1022446871287307213, 0.1041013232007219902, 0.1050296412367176246, 0.1054938002547154419, 0.1059579592727132452, 0.1064221182907110486, 0.1068862773087088658, 0.1078145953447045002, 0.1096712314166957691, 0.1105995494526914036, 0.1115278674886870380, 0.1124561855246826725, 0.1133845035606783069, 0.1143128215966739414, 0.1152411396326695758, 0.1170977757046608447, 0.1180260937406564792, 0.1184902527586542964, 0.1189544117766521136, 0.1194185707946499309, 0.1198827298126477481, 0.1208110478486433687 ),
 .UNSPECIFIED. ) ;
#17425=CARTESIAN_POINT ( 'NONE',  ( 199.9999999999999147, 0.6045081272180472531, 19.00173049909658474 ) ) ;
#17456=CARTESIAN_POINT ( 'NONE',  ( 199.0248560840425682, -19.46388604182612880, 4.665080622506349251 ) ) ;
#17464=CARTESIAN_POINT ( 'NONE',  ( 0.2972598230769959993, 38.42060263243713081, -38.42060263243619289 ) ) ;
#17466=CARTESIAN_POINT ( 'NONE',  ( 199.9999999999999432, -6.993216068016765874, -17.67234381275832433 ) ) ;
#17478=CARTESIAN_POINT ( 'NONE',  ( 130.8568914410475372, -24.07718906447255947, 24.07718906447199458 ) ) ;
#17491=CARTESIAN_POINT ( 'NONE',  ( 199.9999999999997726, -8.411091645968788555, 17.05096182211362432 ) ) ;
#17518=CARTESIAN_POINT ( 'NONE',  ( 200.0000000000000568, 2.630809070280605511, -18.81871160794394982 ) ) ;
#17522=CARTESIAN_POINT ( 'NONE',  ( 199.0070875033960078, 19.58406838943379569, -4.039067077891903779 ) ) ;
#17528=CARTESIAN_POINT ( 'NONE',  ( 199.0053211804427633, 14.13331159297750617, -14.14343255912447361 ) ) ;
#17540=CARTESIAN_POINT ( 'NONE',  ( -91.56559293963834989, -16.03295912088728414, 16.03295912088688269 ) ) ;
#17548=VERTEX_POINT ( 'NONE', #22719 ) ;
#17550=CARTESIAN_POINT ( 'NONE',  ( 200.0000000000000568, -6.707298731100607370, 17.79007541258576452 ) ) ;
#17580=CARTESIAN_POINT ( 'NONE',  ( 199.0250265424592726, -19.30222243252582714, 5.292048582057746309 ) ) ;
#17587=CARTESIAN_POINT ( 'NONE',  ( -91.56559293963834989, 12.25131212657497848, -12.25131212657469426 ) ) ;
#17589=CARTESIAN_POINT ( 'NONE',  ( 199.9999999999998295, -18.94756416210704941, 1.560766781390804381 ) ) ;
#17616=CARTESIAN_POINT ( 'NONE',  ( 199.9999999999998010, -6.124229907523811356, 17.99904841416608292 ) ) ;
#17643=CARTESIAN_POINT ( 'NONE',  ( 199.9999999999998863, -15.98179559645994097, -10.29177186004950961 ) ) ;
#17646=CARTESIAN_POINT ( 'NONE',  ( 199.0054653064281922, 16.25946365448332998, -11.63817148238572940 ) ) ;
#17677=CARTESIAN_POINT ( 'NONE',  ( 200.0000000000001421, -10.70065846580424207, 15.71346033962178446 ) ) ;
#17710=CARTESIAN_POINT ( 'NONE',  ( 199.0159014060021150, -14.06460796087901954, -14.21930665748418576 ) ) ;
#17719=CARTESIAN_POINT ( 'NONE',  ( -105.3755690713226727, 12.89780903124418998, -12.89780903124389155 ) ) ;
#17722=CARTESIAN_POINT ( 'NONE',  ( 199.9999999999999432, -17.61942792365240607, -7.131405496535110800 ) ) ;
#17749=CARTESIAN_POINT ( 'NONE',  ( 200.0000000000000000, 12.97704027674654270, 13.88623514161034045 ) ) ;
#17763=CARTESIAN_POINT ( 'NONE',  ( 200.0000000000000000, 14.14213562373041455, 42.42640687119311593 ) ) ;
#17766=FACE_OUTER_BOUND ( 'NONE', #21084, .T. ) ;
#17775=CARTESIAN_POINT ( 'NONE',  ( 200.0000000000002274, -16.15590588650048787, 10.03807108387658786 ) ) ;
#17778=CARTESIAN_POINT ( 'NONE',  ( 199.0066757862822726, 19.23093628729661475, -5.478378800400602877 ) ) ;
#17797=CARTESIAN_POINT ( 'NONE',  ( 136.1360204305621266, -24.77266263493151044, 24.77266263493093135 ) ) ;
#17808=CARTESIAN_POINT ( 'NONE',  ( 199.9999999999996305, 13.20330696038688068, 13.67115712520468840 ) ) ;
#17814=CARTESIAN_POINT ( 'NONE',  ( 14.38125909742181108, 39.01709431150961649, -39.01709431150867147 ) ) ;
#17819=EDGE_CURVE ( 'NONE', #8765, #17548, #18475, .T. ) ;
#17823=CARTESIAN_POINT ( 'NONE',  ( -280.0000000000000000, 9.999999999999948486, 1.224646799147346354E-15 ) ) ;
#17850=CARTESIAN_POINT ( 'NONE',  ( -213.1075012329537230, 37.98287015391280619, -37.98287015391192512 ) ) ;
#17853=CARTESIAN_POINT ( 'NONE',  ( 199.0142490642952566, 16.24935999037262846, 11.66321269349018941 ) ) ;
#17866=CARTESIAN_POINT ( 'NONE',  ( 199.9999999999999432, -14.14213562373115884, 14.14213562373085153 ) ) ;
#17880=PLANE ( 'NONE',  #13415 ) ;
#17881=CARTESIAN_POINT ( 'NONE',  ( 199.9999999999996021, 18.99368777275013898, 0.6330478706754758544 ) ) ;
#17882=CARTESIAN_POINT ( 'NONE',  ( 199.9999999999999147, -9.234286251058666295, -16.61017430452723787 ) ) ;
#17894=CARTESIAN_POINT ( 'NONE',  ( 146.6084372240433709, 3.800685668858042821, 52.76785682606522698 ) ) ;
#17897=CARTESIAN_POINT ( 'NONE',  ( -259.2033419157646676, 21.55415060305790931, 35.01439189186571355 ) ) ;
#17914=CARTESIAN_POINT ( 'NONE',  ( 199.0064300139308102, 18.94043123351016433, -6.416860702434988184 ) ) ;
#17942=CARTESIAN_POINT ( 'NONE',  ( 200.0000000000000568, 16.12943746570313053, 10.05448153537135347 ) ) ;
#17948=CARTESIAN_POINT ( 'NONE',  ( 130.8568914410475372, 4.207082182992923691, -4.207082182992794017 ) ) ;
#17973=CARTESIAN_POINT ( 'NONE',  ( 200.0000000000000000, 18.50924455979920324, -4.296878913645367781 ) ) ;
#17979=CARTESIAN_POINT ( 'NONE',  ( 199.0079861221352360, 1.294590733001960592, -19.95474696286750671 ) ) ;
#17986=CARTESIAN_POINT ( 'NONE',  ( 199.0135736376541615, 16.97384353125803003, 10.58053792802146020 ) ) ;
#18016=CARTESIAN_POINT ( 'NONE',  ( 199.9999999999998579, 13.86282612285610938, 13.00154682524819805 ) ) ;
#18017=CARTESIAN_POINT ( 'NONE',  ( 199.9999999999999716, -16.91202053066619371, 8.687169125204889042 ) ) ;
#18027=CARTESIAN_POINT ( 'NONE',  ( 199.0263771133097350, -13.25980953972711340, 15.03167181779690331 ) ) ;
#18028=CARTESIAN_POINT ( 'NONE',  ( -208.1127848780265026, 38.89260858015777700, -38.89260858015687461 ) ) ;
#18031=CARTESIAN_POINT ( 'NONE',  ( 130.8568914410475372, -24.07718906447255947, 24.07718906447199458 ) ) ;
#18041=CARTESIAN_POINT ( 'NONE',  ( 199.9999999999998579, -17.68075590865577951, 6.990562776172230208 ) ) ;
#18046=CARTESIAN_POINT ( 'NONE',  ( 199.0191706476670959, -17.79509468669765226, -9.138050845474172235 ) ) ;
#18068=EDGE_LOOP ( 'NONE', ( #5455, #21425 ) ) ;
#18076=CARTESIAN_POINT ( 'NONE',  ( 200.0000000000000568, 7.542793502284206753, 17.44923311141863920 ) ) ;
#18084=CARTESIAN_POINT ( 'NONE',  ( -91.56559293963834989, -16.03295912088659492, -40.53558337403696044 ) ) ;
#18085=CARTESIAN_POINT ( 'NONE',  ( 199.0231121918538975, 0.6363371645724309467, 19.99606429142543362 ) ) ;
#18110=CARTESIAN_POINT ( 'NONE',  ( 199.9999999999999432, 18.69211761857796361, 3.422848245100247766 ) ) ;
#18117=CARTESIAN_POINT ( 'NONE',  ( 199.0097193260481561, -3.097360908056462137, -19.75623422735097989 ) ) ;
#18125=CARTESIAN_POINT ( 'NONE',  ( 199.0163148259956358, 13.65645126726637670, 14.61284818176725331 ) ) ;
#18152=CARTESIAN_POINT ( 'NONE',  ( 200.0000000000000284, 17.23849352212496910, 7.999418879479941680 ) ) ;
#18154=CARTESIAN_POINT ( 'NONE',  ( 199.9999999999999147, -18.75789134796499624, 3.098008012732793137 ) ) ;
#18164=CARTESIAN_POINT ( 'NONE',  ( 199.0255398360378365, -7.415439759742569414, 18.57980843913382429 ) ) ;
#18165=CARTESIAN_POINT ( 'NONE',  ( -192.9588430854689989, 38.51493924976983152, -38.51493924976893624 ) ) ;
#18167=CARTESIAN_POINT ( 'NONE',  ( -105.3755690713226727, -15.38646221621807619, 15.38646221621768362 ) ) ;
#18176=CARTESIAN_POINT ( 'NONE',  ( 199.9999999999999716, -17.31617203886849410, 7.850475485701642775 ) ) ;
#18180=CARTESIAN_POINT ( 'NONE',  ( 199.0138211924391385, -10.98290011267725141, -16.71408225681557980 ) ) ;
#18205=CARTESIAN_POINT ( 'NONE',  ( 200.0000000000002558, 14.28373528157942829, 12.54030857537068755 ) ) ;
#18211=CARTESIAN_POINT ( 'NONE',  ( 192.4448373802101173, -14.14213562375826605, -42.42640687116518450 ) ) ;
#18212=CARTESIAN_POINT ( 'NONE',  ( 199.0260893535204048, -10.43036187021208860, 17.07141274968551059 ) ) ;
#18240=CARTESIAN_POINT ( 'NONE',  ( 199.9999999999998863, 18.97030179798468907, 1.258860953597385590 ) ) ;
#18247=CARTESIAN_POINT ( 'NONE',  ( 199.0140770886559949, -11.39180206020552788, -16.43826011434489587 ) ) ;
#18255=CARTESIAN_POINT ( 'NONE',  ( 199.9999999999996589, -18.76526504493254777, 3.099636891498418478 ) ) ;
#18258=CARTESIAN_POINT ( 'NONE',  ( 199.0227319893622848, 1.617020328492027259, 19.94056979940310015 ) ) ;
#18284=CARTESIAN_POINT ( 'NONE',  ( 200.0000000000000000, 15.44098642598172866, 11.08330662512073950 ) ) ;
#18285=CARTESIAN_POINT ( 'NONE',  ( 199.9999999999999147, -15.72534676981639201, 10.68315640806297040 ) ) ;
#18294=CARTESIAN_POINT ( 'NONE',  ( 199.0196953583521520, 8.175823868318582655, 18.25500783319687415 ) ) ;
#18295=CARTESIAN_POINT ( 'NONE',  ( 91.82158438592158234, 44.40256751092319121, 12.16597498400105515 ) ) ;
#18297=CARTESIAN_POINT ( 'NONE',  ( -30.26275506840325136, 57.76657404653985139, -1.198031551615314161 ) ) ;
#18305=ORIENTED_EDGE ( 'NONE', *, *, #11113, .F. ) ;
#18311=CARTESIAN_POINT ( 'NONE',  ( 199.9999999999998863, -16.91159699891635171, 8.687942971654136315 ) ) ;
#18314=CARTESIAN_POINT ( 'NONE',  ( 199.0078712948245823, 1.622169390422157242, -19.93073376281416031 ) ) ;
#18346=CARTESIAN_POINT ( 'NONE',  ( 199.9999999999998579, 17.43084440603007224, 7.570815656493459223 ) ) ;
#18353=CARTESIAN_POINT ( 'NONE',  ( -198.0356074513804572, 10.87444709761036066, -67.44298959253325165 ) ) ;
#18354=CARTESIAN_POINT ( 'NONE',  ( 199.0252416244725282, -6.134786337322394090, 19.04345623536530141 ) ) ;
#18380=CARTESIAN_POINT ( 'NONE',  ( 199.9999999999999716, 18.60999626737240931, -3.837347524953120370 ) ) ;
#18385=CARTESIAN_POINT ( 'NONE',  ( 199.0059805750804571, 8.391908656364034158, -18.14947886101857932 ) ) ;
#18395=CARTESIAN_POINT ( 'NONE',  ( 199.0188463327468185, 9.707946089746242180, 17.48826952134088941 ) ) ;
#18421=CARTESIAN_POINT ( 'NONE',  ( 200.0000000000002274, 18.09557305485218848, -5.802546270622393365 ) ) ;
#18422=CARTESIAN_POINT ( 'NONE',  ( 199.9999999999999716, -17.68120445620925096, 6.989503635265373660 ) ) ;
#18425=B_SPLINE_CURVE_WITH_KNOTS ( 'NONE', 3,
 ( #12185, #18027, #9921, #2216, #16306, #6196, #4350, #1950, #15893, #18164, #10325, #6322, #2083, #22307, #16170, #12048, #209, #13907, #14043, #5800, #24305, #24430, #24567, #22177, #22041, #6072, #26176, #11918, #7917, #3951, #20306, #4084, #8190, #14174, #80, #10190, #20168, #14443, #20040, #10057, #18294, #5936, #2343, #22572, #16034, #12442, #14309, #4221, #12311, #20438, #18433, #24159, #20570, #7778, #24021, #3814, #1818, #14834, #616, #6722, #10726, #23105, #21103, #15097, #20838, #883, #8993, #6456, #4476, #16570, #2750, #2474, #22966, #18837, #17097, #3007, #4746, #12852, #14571, #14970, #24973, #24701, #22701, #10854, #16701, #8722, #25104, #752, #20708, #2613, #4614, #23230, #5008, #8856, #2883, #24833, #18700, #13113, #16840, #14706, #6853, #10991, #16968, #4877 ),
 .UNSPECIFIED., .F., .F.,
 ( 4, 2, 2, 2, 1, 1, 1, 2, 2, 2, 2, 2, 1, 1, 1, 1, 2, 2, 2, 2, 2, 1, 1, 1, 1, 1, 2, 2, 2, 2, 2, 2, 1, 1, 2, 2, 2, 2, 2, 2, 1, 1, 1, 1, 2, 2, 2, 2, 2, 1, 1, 1, 2, 2, 2, 2, 2, 1, 1, 1, 2, 2, 2, 4 ),
 ( 0.000000000000000000, 0.03124629074579460611, 0.06249258149158921222, 0.06298080478449225028, 0.06346902807739529528, 0.06444547466320135753, 0.06639836783481350979, 0.07030415417803781430, 0.07811572686448636782, 0.09373887223738347485, 0.1249851629831776750, 0.1252292746296291837, 0.1254733862760807062, 0.1259616095689837512, 0.1269380561547898412, 0.1288909493264019657, 0.1327967356696262424, 0.1406083083560747959, 0.1562314537289719030, 0.1874777444747661170, 0.1875998002979918367, 0.1877218561212175840, 0.1879659677676691343, 0.1884541910605721793, 0.1894306376463783248, 0.1913835308179905881, 0.1952893171612150591, 0.2031008898476640012, 0.2187240352205620242, 0.2343471805934600194, 0.2499703259663580701, 0.2509467725521641879, 0.2519232191379703334, 0.2538761123095825689, 0.2577818986528070400, 0.2655934713392559821, 0.2812166167121538107, 0.2968397620850516949, 0.3124629074579495791, 0.3127070191044010739, 0.3129511307508526241, 0.3134393540437556136, 0.3144158006295616481, 0.3163686938011737171, 0.3202744801443978551, 0.3280860528308460755, 0.3437091982037425719, 0.3749554889495356758, 0.3754437122424387208, 0.3759319355353417658, 0.3769083821211477447, 0.3788612752927598137, 0.3827670616359840072, 0.3905786343224322832, 0.4062017796953287796, 0.4374480704411218279, 0.4379362937340248729, 0.4384245170269279179, 0.4394009636127340634, 0.4413538567843462990, 0.4452596431275708810, 0.4530712158140199342, 0.4686943611869179849, 0.4999406519327141418 ),
 .UNSPECIFIED. ) ;
#18426=DIRECTION ( 'NONE',  ( 1.298934084353256076E-16, -0.7071067811865561215, 0.7071067811865389130 ) ) ;
#18433=CARTESIAN_POINT ( 'NONE',  ( 199.0159127812860049, 14.20410482617004710, 14.07996899236659871 ) ) ;
#18435=CARTESIAN_POINT ( 'NONE',  ( -30.26275506840323715, 29.48230279907829754, -29.48230279907758344 ) ) ;
#18437=CARTESIAN_POINT ( 'NONE',  ( -238.4067589809705794, 57.25054294065799354, -0.6820004457334954973 ) ) ;
#18448=CARTESIAN_POINT ( 'NONE',  ( 199.0102239786929488, -4.226749394367478097, -19.54603893341629473 ) ) ;
#18475=B_SPLINE_CURVE_WITH_KNOTS ( 'NONE', 1,
 ( #17528, #13792 ),
 .UNSPECIFIED., .F., .F.,
 ( 2, 2 ),
 ( 0.000000000000000000, 1.000000000000000000 ),
 .UNSPECIFIED. ) ;
#18476=CARTESIAN_POINT ( 'NONE',  ( 199.9999999999998010, 4.312122466882670757, -18.50761716938983525 ) ) ;
#18482=CARTESIAN_POINT ( 'NONE',  ( -213.1075012329537230, 9.698598906450543566, -9.698598906450348167 ) ) ;
#18483=CARTESIAN_POINT ( 'NONE',  ( 199.0255290512018291, -7.361955815226616906, 18.60363316911454845 ) ) ;
#18511=CARTESIAN_POINT ( 'NONE',  ( 199.9999999999999716, 10.29099968577115654, 15.98230674020753206 ) ) ;
#18517=CARTESIAN_POINT ( 'NONE',  ( 199.0058364129993436, 9.132953877242854901, -17.78802470895853816 ) ) ;
#18530=CARTESIAN_POINT ( 'NONE',  ( 199.0053384867209445, 15.04244419640346031, -13.18878631234924192 ) ) ;
#18558=CARTESIAN_POINT ( 'NONE',  ( 200.0000000000002558, 2.008769787671115026, -18.89534854373681938 ) ) ;
#18559=CARTESIAN_POINT ( 'NONE',  ( 199.9999999999999432, 6.970163742134758422, -17.67854661859792031 ) ) ;
#18569=CARTESIAN_POINT ( 'NONE',  ( 163.1118516004056573, 37.29075403953132906, 19.27778845539275565 ) ) ;
#18571=CARTESIAN_POINT ( 'NONE',  ( 200.0000000000000000, 14.14213562373041455, 42.42640687119311593 ) ) ;
#18575=VECTOR ( 'NONE', #2072, 1000.000000000000000 ) ;
#18588=CARTESIAN_POINT ( 'NONE',  ( 199.0140770886559949, -11.39180206020552788, -16.43826011434489587 ) ) ;
#18613=CARTESIAN_POINT ( 'NONE',  ( 200.0000000000000853, 3.093441846007485285, -18.74813587279223981 ) ) ;
#18620=CARTESIAN_POINT ( 'NONE',  ( -30.26275506840324070, -27.08623969584554558, -29.48230279907826912 ) ) ;
#18621=CARTESIAN_POINT ( 'NONE',  ( 199.0248237628271113, -4.554872532684343334, 19.47958378538321611 ) ) ;
#18644=CARTESIAN_POINT ( 'NONE',  ( 199.9999999999999147, -12.54556961440541585, 14.29646200777123788 ) ) ;
#18650=CARTESIAN_POINT ( 'NONE',  ( 199.0203632001705216, -18.77805633539013996, -6.891912269405206182 ) ) ;
#18660=CARTESIAN_POINT ( 'NONE',  ( 199.0076515966382260, 19.86999350167783263, -2.263549309587763680 ) ) ;
#18675=CARTESIAN_POINT ( 'NONE',  ( 199.0148543684761080, -12.57771741307266744, -15.55405153308071320 ) ) ;
#18689=CARTESIAN_POINT ( 'NONE',  ( 200.0000000000000284, 8.678546691382686973, -16.90316441639222944 ) ) ;
#18690=CARTESIAN_POINT ( 'NONE',  ( 199.9999999999999716, 6.098650052811386502, -17.99789284726596961 ) ) ;
#18700=CARTESIAN_POINT ( 'NONE',  ( 199.0059807619071535, 18.14866951045441112, -8.393696149220648550 ) ) ;
#18702=CARTESIAN_POINT ( 'NONE',  ( 4.995406935893294431, -17.50105314357144337, -39.06748935135212264 ) ) ;
#18704=CARTESIAN_POINT ( 'NONE',  ( -91.56559293963834989, 12.25131212657428748, 44.31723036834913643 ) ) ;
#18716=CARTESIAN_POINT ( 'NONE',  ( 199.0250768083106436, -19.24006491846622069, 5.486913247009519878 ) ) ;
#18748=CARTESIAN_POINT ( 'NONE',  ( 199.9999999999999147, 19.00141375156598045, 0.3223421948013435179 ) ) ;
#18751=CARTESIAN_POINT ( 'NONE',  ( 91.82158438592158234, -40.45024623143936537, -16.11829626348475131 ) ) ;
#18752=CARTESIAN_POINT ( 'NONE',  ( 199.0095182511445557, 19.82538855659994681, 2.633105091475395287 ) ) ;
#18767=CARTESIAN_POINT ( 'NONE',  ( 199.0263771353516233, -14.14574067859894413, 14.14574067859863682 ) ) ;
#18781=CARTESIAN_POINT ( 'NONE',  ( 199.9999999999999147, 1.227885840012788776, 18.97153672786391709 ) ) ;
#18789=CARTESIAN_POINT ( 'NONE',  ( 199.0143331921596257, -11.79252763263196613, -16.15335214697885391 ) ) ;
#18801=CARTESIAN_POINT ( 'NONE',  ( 199.0069448139248891, 19.47830345430216070, -4.521371627647083891 ) ) ;
#18815=CARTESIAN_POINT ( 'NONE',  ( 199.0119081132318115, -7.641483972870305230, -18.48045621412796891 ) ) ;
#18825=CARTESIAN_POINT ( 'NONE',  ( 199.9999999999998010, -4.930716969832944940, -18.35446462305003834 ) ) ;
#18832=B_SPLINE_CURVE_WITH_KNOTS ( 'NONE', 1,
 ( #25713, #3355 ),
 .UNSPECIFIED., .F., .F.,
 ( 2, 2 ),
 ( 0.000000000000000000, 1.000000000000000000 ),
 .UNSPECIFIED. ) ;
#18837=CARTESIAN_POINT ( 'NONE',  ( 199.0105800778188723, 19.37561348799876626, 4.995799333890384553 ) ) ;
#18839=CARTESIAN_POINT ( 'NONE',  ( -56.48582580120559982, -34.75652343174584047, -21.81201906317815187 ) ) ;
#18853=CARTESIAN_POINT ( 'NONE',  ( 199.0220583073800640, -19.74674823417053915, -3.257374120286249397 ) ) ;
#18881=CARTESIAN_POINT ( 'NONE',  ( 199.9999999999999716, 7.832101404672591194, -17.31171755797958056 ) ) ;
#18885=CARTESIAN_POINT ( 'NONE',  ( 136.1360204305621266, -24.77266263493151044, 24.77266263493093135 ) ) ;
#18886=CARTESIAN_POINT ( 'NONE',  ( 199.0168302869249999, 12.92424399662411005, 15.26720349029574564 ) ) ;
#18913=CARTESIAN_POINT ( 'NONE',  ( 199.9999999999999716, -10.04560847499968368, 16.14005499122785281 ) ) ;
#18919=CARTESIAN_POINT ( 'NONE',  ( 199.0249934254769926, -19.32713910159323589, 5.171593721336591010 ) ) ;
#18933=CARTESIAN_POINT ( 'NONE',  ( 199.0112867096082141, 18.93484222638594616, 6.440921653838688421 ) ) ;
#18950=CARTESIAN_POINT ( 'NONE',  ( 199.0055949646623503, 10.60095110936554974, -16.96607438669680334 ) ) ;
#18962=CARTESIAN_POINT ( 'NONE',  ( 200.0000000000003126, 15.08009544811998204, -11.56244146370294779 ) ) ;
#18973=CARTESIAN_POINT ( 'NONE',  ( -86.96347745069644475, -15.38646221621807442, 15.38646221621768184 ) ) ;
#18989=CARTESIAN_POINT ( 'NONE',  ( 199.0238156666156044, -19.96322609118500324, 1.315852278599464631 ) ) ;
#19017=CARTESIAN_POINT ( 'NONE',  ( 200.0000000000001421, 16.62132632430557777, -9.210632111445709924 ) ) ;
#19020=CARTESIAN_POINT ( 'NONE',  ( -86.96347745069644475, -43.67073346367964604, -12.89780903124457545 ) ) ;
#19021=CARTESIAN_POINT ( 'NONE',  ( 199.0158819412750688, 14.24569456864689343, 14.03872682698725249 ) ) ;
#19051=CARTESIAN_POINT ( 'NONE',  ( 199.0152737994447136, -13.19951906643276374, -15.03942049639883294 ) ) ;
#19062=CARTESIAN_POINT ( 'NONE',  ( 199.0054122081438948, 15.86953797770180508, -12.16778084942700211 ) ) ;
#19080=CARTESIAN_POINT ( 'NONE',  ( 199.0084611626479045, -0.003522264206503993803, -19.99626311085798136 ) ) ;
#19092=CARTESIAN_POINT ( 'NONE',  ( 199.9999999999999432, 15.63063699308155030, -10.80328371702407786 ) ) ;
#19093=CARTESIAN_POINT ( 'NONE',  ( 199.9999999999999432, -0.3235039025349020214, -19.00140615985569070 ) ) ;
#19101=CARTESIAN_POINT ( 'NONE',  ( 200.0000000000000000, -42.42640687119272513, -14.14213562373140753 ) ) ;
#19115=CARTESIAN_POINT ( 'NONE',  ( 200.0000000000003695, -13.00390091431020956, 13.88089034683036616 ) ) ;
#19141=CARTESIAN_POINT ( 'NONE',  ( 200.0000000000001137, 2.164978928433492822, -18.87806096587463855 ) ) ;
#19145=CARTESIAN_POINT ( 'NONE',  ( 199.0106735244355320, 19.32142130491951804, 5.196343561012195522 ) ) ;
#19159=CARTESIAN_POINT ( 'NONE',  ( 199.0253172846266523, -6.444568167316012008, 18.94088585829734228 ) ) ;
#19161=CARTESIAN_POINT ( 'NONE',  ( 19.06497207195979726, 38.31983398719604139, 18.24870850772803976 ) ) ;
#19179=CARTESIAN_POINT ( 'NONE',  ( 199.0253131443098766, -18.94683372192476156, 6.427280041807147626 ) ) ;
#19208=CARTESIAN_POINT ( 'NONE',  ( 199.0082391558451320, 0.5918947795737343753, -19.98868739452279897 ) ) ;
#19213=UNCERTAINTY_MEASURE_WITH_UNIT (LENGTH_MEASURE( 1.000000000000000082E-05 ), #10268, 'distance_accuracy_value', 'NONE');
#19215=EDGE_CURVE ( 'NONE', #13305, #15869, #18425, .T. ) ;
#19219=CARTESIAN_POINT ( 'NONE',  ( 199.9999999999999432, -14.29115147104986860, -12.53286550942210198 ) ) ;
#19230=CARTESIAN_POINT ( 'NONE',  ( 91.82158438592158234, -12.16597498399995203, -44.40256751092347542 ) ) ;
#19244=CARTESIAN_POINT ( 'NONE',  ( 199.9999999999996589, -3.408648353384132079, 18.70401797595889448 ) ) ;
#19260=DIRECTION ( 'NONE',  ( -1.000000000000000000, -1.836970198721030181E-16, -2.465190328815661892E-32 ) ) ;
#19269=CARTESIAN_POINT ( 'NONE',  ( 199.9999999999998295, 1.074487055219422560, -18.97158139261448540 ) ) ;
#19272=CARTESIAN_POINT ( 'NONE',  ( 199.0097993503064515, 19.72850438885342328, 3.281923459752313921 ) ) ;
#19286=CARTESIAN_POINT ( 'NONE',  ( 146.6084372240433993, -24.48358557860353457, 24.48358557860296258 ) ) ;
#19301=CARTESIAN_POINT ( 'NONE',  ( 200.0000000000001421, -0.6349535514222880428, 19.00853270881595591 ) ) ;
#19316=( BOUNDED_SURFACE ( )  B_SPLINE_SURFACE ( 3, 3, ( 
 ( #815, #22899, #12780, #6265, #4289, #12378, #20506, #8386, #4413, #11171, #2940, #3541, #7171, #13174, #19763, #1069, #15288, #13771, #6917, #15167, #5801, #17289, #11641, #19286, #24022, #4943, #11783, #1687, #25166, #13049 ),
 ( #23292, #21295, #13908, #3069, #25423, #15034, #20041, #9178, #23418, #5536, #15895, #21167, #13642, #11050, #23164, #21898, #7050, #3675, #19161, #1554, #21768, #19903, #9791, #17894, #946, #9659, #8921, #26042, #9054, #17763 ),
 ( #11919, #17159, #7779, #25905, #25293, #22043, #5068, #7646, #15760, #3816, #17031, #23889, #5665, #6324, #14310, #12050, #2344, #10059, #2217, #24431, #18295, #8319, #16572, #22309, #10456, #18569, #24306, #349, #24568, #1951 ),
 ( #14446, #22178, #16444, #26312, #18028, #8191, #18165, #10326, #24703, #14044, #81, #8055, #10192, #14175, #18435, #210, #3952, #4085, #6073, #14573, #16171, #5937, #8453, #16307, #22702, #12186, #20308, #22573, #6457, #4477 ),
 ( #4351, #12579, #2085, #6198, #12443, #22444, #4224, #12313, #20439, #20572, #1820, #9922, #26178, #7918, #16035, #24161, #20169, #485, #25363, #25231, #19230, #4747, #17098, #6983, #12853, #15098, #2884, #7118, #14707, #15228 ),
 ( #617, #17224, #2752, #23106, #20971, #9113, #16702, #23232, #13114, #10587, #24834, #6586, #5136, #18839, #23359, #8857, #18702, #20709, #8723, #22968, #8592, #2614, #22840, #5009, #4615, #2475, #3009, #12711, #21235, #19101 ),
 ( #12982, #10855, #11116, #1010, #20839, #10727, #6723, #16841, #24974, #14835, #10992, #885, #18973, #753, #16969, #25105, #6854, #14971, #4878, #21104, #8994, #17478, #7366, #3648, #15604, #5510, #21482, #1526, #19354, #17866 ) ),
 .UNSPECIFIED., .T., .F., .T. ) 
 B_SPLINE_SURFACE_WITH_KNOTS ( ( 4, 3, 4 ),
 ( 4, 2, 2, 2, 2, 2, 2, 2, 2, 2, 2, 2, 2, 2, 4 ),
 ( 0.000000000000000000, 0.5000000000000000000, 1.000000000000000000 ),
 ( 0.000000000000000000, 0.1357259735107005372, 0.1651108541090157700, 0.1944957347073310028, 0.3598804999793158710, 0.3867117631979620773, 0.4135430264166082281, 0.5789277916885930964, 0.6062785021374117456, 0.6336292125862302838, 0.8508620842112317728, 0.8814014469398914198, 0.9119408096685510667, 0.9559704048342755334, 1.000000000000000000 ),
 .UNSPECIFIED. ) 
 GEOMETRIC_REPRESENTATION_ITEM ( )  RATIONAL_B_SPLINE_SURFACE ( (
 ( 1.000000000000000000, 1.000000000000000000, 1.000000000000000000, 1.000000000000000000, 1.000000000000000000, 1.000000000000000000, 1.000000000000000000, 1.000000000000000000, 1.000000000000000000, 1.000000000000000000, 1.000000000000000000, 1.000000000000000000, 1.000000000000000000, 1.000000000000000000, 1.000000000000000000, 1.000000000000000000, 1.000000000000000000, 1.000000000000000000, 1.000000000000000000, 1.000000000000000000, 1.000000000000000000, 1.000000000000000000, 1.000000000000000000, 1.000000000000000000, 1.000000000000000000, 1.000000000000000000, 1.000000000000000000, 1.000000000000000000, 1.000000000000000000, 1.000000000000000000),
 ( 0.3333333333333333703, 0.3333333333333333703, 0.3333333333333333703, 0.3333333333333333703, 0.3333333333333333703, 0.3333333333333333703, 0.3333333333333333703, 0.3333333333333333703, 0.3333333333333333703, 0.3333333333333333703, 0.3333333333333333703, 0.3333333333333333703, 0.3333333333333333703, 0.3333333333333333703, 0.3333333333333333703, 0.3333333333333333703, 0.3333333333333333703, 0.3333333333333333703, 0.3333333333333333703, 0.3333333333333333703, 0.3333333333333333703, 0.3333333333333333703, 0.3333333333333333703, 0.3333333333333333703, 0.3333333333333333703, 0.3333333333333333703, 0.3333333333333333703, 0.3333333333333333703, 0.3333333333333333703, 0.3333333333333333703),
 ( 0.3333333333333333703, 0.3333333333333333703, 0.3333333333333333703, 0.3333333333333333703, 0.3333333333333333703, 0.3333333333333333703, 0.3333333333333333703, 0.3333333333333333703, 0.3333333333333333703, 0.3333333333333333703, 0.3333333333333333703, 0.3333333333333333703, 0.3333333333333333703, 0.3333333333333333703, 0.3333333333333333703, 0.3333333333333333703, 0.3333333333333333703, 0.3333333333333333703, 0.3333333333333333703, 0.3333333333333333703, 0.3333333333333333703, 0.3333333333333333703, 0.3333333333333333703, 0.3333333333333333703, 0.3333333333333333703, 0.3333333333333333703, 0.3333333333333333703, 0.3333333333333333703, 0.3333333333333333703, 0.3333333333333333703),
 ( 1.000000000000000000, 1.000000000000000000, 1.000000000000000000, 1.000000000000000000, 1.000000000000000000, 1.000000000000000000, 1.000000000000000000, 1.000000000000000000, 1.000000000000000000, 1.000000000000000000, 1.000000000000000000, 1.000000000000000000, 1.000000000000000000, 1.000000000000000000, 1.000000000000000000, 1.000000000000000000, 1.000000000000000000, 1.000000000000000000, 1.000000000000000000, 1.000000000000000000, 1.000000000000000000, 1.000000000000000000, 1.000000000000000000, 1.000000000000000000, 1.000000000000000000, 1.000000000000000000, 1.000000000000000000, 1.000000000000000000, 1.000000000000000000, 1.000000000000000000),
 ( 0.3333333333333333703, 0.3333333333333333703, 0.3333333333333333703, 0.3333333333333333703, 0.3333333333333333703, 0.3333333333333333703, 0.3333333333333333703, 0.3333333333333333703, 0.3333333333333333703, 0.3333333333333333703, 0.3333333333333333703, 0.3333333333333333703, 0.3333333333333333703, 0.3333333333333333703, 0.3333333333333333703, 0.3333333333333333703, 0.3333333333333333703, 0.3333333333333333703, 0.3333333333333333703, 0.3333333333333333703, 0.3333333333333333703, 0.3333333333333333703, 0.3333333333333333703, 0.3333333333333333703, 0.3333333333333333703, 0.3333333333333333703, 0.3333333333333333703, 0.3333333333333333703, 0.3333333333333333703, 0.3333333333333333703),
 ( 0.3333333333333333703, 0.3333333333333333703, 0.3333333333333333703, 0.3333333333333333703, 0.3333333333333333703, 0.3333333333333333703, 0.3333333333333333703, 0.3333333333333333703, 0.3333333333333333703, 0.3333333333333333703, 0.3333333333333333703, 0.3333333333333333703, 0.3333333333333333703, 0.3333333333333333703, 0.3333333333333333703, 0.3333333333333333703, 0.3333333333333333703, 0.3333333333333333703, 0.3333333333333333703, 0.3333333333333333703, 0.3333333333333333703, 0.3333333333333333703, 0.3333333333333333703, 0.3333333333333333703, 0.3333333333333333703, 0.3333333333333333703, 0.3333333333333333703, 0.3333333333333333703, 0.3333333333333333703, 0.3333333333333333703),
 ( 1.000000000000000000, 1.000000000000000000, 1.000000000000000000, 1.000000000000000000, 1.000000000000000000, 1.000000000000000000, 1.000000000000000000, 1.000000000000000000, 1.000000000000000000, 1.000000000000000000, 1.000000000000000000, 1.000000000000000000, 1.000000000000000000, 1.000000000000000000, 1.000000000000000000, 1.000000000000000000, 1.000000000000000000, 1.000000000000000000, 1.000000000000000000, 1.000000000000000000, 1.000000000000000000, 1.000000000000000000, 1.000000000000000000, 1.000000000000000000, 1.000000000000000000, 1.000000000000000000, 1.000000000000000000, 1.000000000000000000, 1.000000000000000000, 1.000000000000000000) ) ) 
 REPRESENTATION_ITEM ( '' )  SURFACE ( )  );
#19330=CARTESIAN_POINT ( 'NONE',  ( 199.0238548747951484, -20.00383568556590674, 1.381665862992945915 ) ) ;
#19342=CARTESIAN_POINT ( 'NONE',  ( 200.0000000000000568, -17.44062545528135999, -7.562669404541021656 ) ) ;
#19354=CARTESIAN_POINT ( 'NONE',  ( 192.4448373802100889, -14.14213562375896061, 14.14213562375865330 ) ) ;
#19370=CARTESIAN_POINT ( 'NONE',  ( 200.0000000000002842, -5.234650960127995134, 18.27551028936266775 ) ) ;
#19385=CARTESIAN_POINT ( 'NONE',  ( -265.0000000000000000, -4.867971026610730343E-14, -6.532754371361504014E-30 ) ) ;
#19399=CARTESIAN_POINT ( 'NONE',  ( 199.9999999999998863, -9.504749071264818383, -16.45922038047892144 ) ) ;
#19403=CARTESIAN_POINT ( 'NONE',  ( 199.0070327355206246, 4.219744681889460836, -19.54794762927634366 ) ) ;
#19429=CARTESIAN_POINT ( 'NONE',  ( 199.0263189878286028, -15.57072488730636017, 12.56115478513486217 ) ) ;
#19434=DIRECTION ( 'NONE',  ( -1.000000000000000000, -1.836970198721030181E-16, -2.465190328815661892E-32 ) ) ;
#19463=CARTESIAN_POINT ( 'NONE',  ( -100.7734535825088358, 12.25131212657497848, -12.25131212657469604 ) ) ;
#19466=CARTESIAN_POINT ( 'NONE',  ( 199.9999999999998863, -15.98179559645994097, -10.29177186004950961 ) ) ;
#19493=CARTESIAN_POINT ( 'NONE',  ( 200.0000000000000284, 7.828075510571024687, 17.32306842307162142 ) ) ;
#19517=CARTESIAN_POINT ( 'NONE',  ( 199.9999999999999716, -5.826418053481885906, -18.09029720167993105 ) ) ;
#19522=CARTESIAN_POINT ( 'NONE',  ( 199.0053905349878107, 15.66748078252780374, -12.42684713134076979 ) ) ;
#19543=CARTESIAN_POINT ( 'NONE',  ( -100.7734535825088358, -16.03295912088728770, 16.03295912088687913 ) ) ;
#19552=CARTESIAN_POINT ( 'NONE',  ( 200.0000000000003695, -13.00390091431020956, 13.88089034683036616 ) ) ;
#19594=CARTESIAN_POINT ( 'NONE',  ( -86.96347745069644475, 12.89780903124419353, -12.89780903124389333 ) ) ;
#19596=CARTESIAN_POINT ( 'NONE',  ( 199.9999999999998863, -18.99932777274695539, 0.6272729670678898195 ) ) ;
#19625=CARTESIAN_POINT ( 'NONE',  ( 199.9999999999998863, -7.850736592177782747, 17.31604939001003274 ) ) ;
#19640=CARTESIAN_POINT ( 'NONE',  ( -208.1127848780265026, 10.60833733269551615, -10.60833733269529766 ) ) ;
#19649=CARTESIAN_POINT ( 'NONE',  ( 200.0000000000000568, -11.58056098922197563, -15.07187815445410806 ) ) ;
#19652=CARTESIAN_POINT ( 'NONE',  ( 199.0056040927672711, 16.99126215759308778, -10.54120702991739122 ) ) ;
#19678=CARTESIAN_POINT ( 'NONE',  ( 199.9999999999999432, -11.20938440123365432, 15.35472082164171326 ) ) ;
#19711=CARTESIAN_POINT ( 'NONE',  ( 199.0263771353515949, -14.14574067859894413, 14.14574067859863682 ) ) ;
#19725=CARTESIAN_POINT ( 'NONE',  ( 199.9999999999998295, -11.08011877867584261, -15.44095579151349185 ) ) ;
#19751=CARTESIAN_POINT ( 'NONE',  ( 199.9999999999996021, 1.536416165433052594, 18.94899354046687279 ) ) ;
#19763=CARTESIAN_POINT ( 'NONE',  ( -30.26275506840324070, 1.198031551616030033, -1.198031551616006496 ) ) ;
#19779=CARTESIAN_POINT ( 'NONE',  ( 199.9999999999998863, -17.44218472118251384, 7.566354988273278792 ) ) ;
#19783=CARTESIAN_POINT ( 'NONE',  ( 199.0065087001378572, 6.107362818253672998, -19.04251412529381327 ) ) ;
#19802=CARTESIAN_POINT ( 'NONE',  ( 199.0263771353515949, -14.14574067859894413, 14.14574067859863682 ) ) ;
#19813=CARTESIAN_POINT ( 'NONE',  ( 200.0000000000000000, 2.625635831523228880, 18.82681798050185051 ) ) ;
#19820=CARTESIAN_POINT ( 'NONE',  ( 192.4448373802101173, 42.42640687116487896, 14.14213562375934075 ) ) ;
#19847=CARTESIAN_POINT ( 'NONE',  ( 199.0164104981701030, -14.74880145479427007, -13.53568457017083659 ) ) ;
#19850=VERTEX_POINT ( 'NONE', #8702 ) ;
#19856=CARTESIAN_POINT ( 'NONE',  ( 19.06497207195981147, 38.31983398719673772, -38.31983398719579981 ) ) ;
#19858=CARTESIAN_POINT ( 'NONE',  ( 200.0000000000002558, -14.49689853580991539, 12.29876589910006857 ) ) ;
#19870=EDGE_CURVE ( 'NONE', #8765, #13305, #16207, .T. ) ;
#19880=CARTESIAN_POINT ( 'NONE',  ( -280.0000000000000000, -5.143516556418885058E-14, -6.902532920683853297E-30 ) ) ;
#19889=CARTESIAN_POINT ( 'NONE',  ( 199.9999999999996305, 13.20330696038688068, 13.67115712520468840 ) ) ;
#19890=CARTESIAN_POINT ( 'NONE',  ( 199.9999999999998863, -14.89105141260043119, -11.81423002201253603 ) ) ;
#19902=CIRCLE ( 'NONE', #8494, 20.00000000000001421 ) ;
#19903=CARTESIAN_POINT ( 'NONE',  ( 130.8568914410475088, 4.207082182989012153, 52.36146031193425188 ) ) ;
#19906=CARTESIAN_POINT ( 'NONE',  ( 146.6084372240433993, -24.48358557860353457, 24.48358557860296258 ) ) ;
#19915=CARTESIAN_POINT ( 'NONE',  ( 199.9999999999997442, -19.00693066143141152, -0.3125757794583984839 ) ) ;
#19919=CARTESIAN_POINT ( 'NONE',  ( 199.0073291892102247, 3.255542347464756681, -19.72957075196997323 ) ) ;
#19945=CARTESIAN_POINT ( 'NONE',  ( 200.0000000000001705, 18.83917254958691601, 2.502331228272203223 ) ) ;
#19951=CARTESIAN_POINT ( 'NONE',  ( 163.1118516004056573, 9.006482792069759213, -9.006482792069505194 ) ) ;
#19980=CARTESIAN_POINT ( 'NONE',  ( 199.9999999999999432, 10.02849973080021684, 16.14841691778726940 ) ) ;
#19986=CARTESIAN_POINT ( 'NONE',  ( 199.0058097323984327, 9.278912463403225175, -17.71230630396810213 ) ) ;
#19995=CARTESIAN_POINT ( 'NONE',  ( 199.0193391886810446, 8.833261569310058903, 17.94623560139499574 ) ) ;
#20029=CARTESIAN_POINT ( 'NONE',  ( 199.9999999999998863, 17.10417011681778732, 8.282922153951966848 ) ) ;
#20030=CARTESIAN_POINT ( 'NONE',  ( 199.9999999999999716, -14.89501297105162969, 11.81655986308013873 ) ) ;
#20040=CARTESIAN_POINT ( 'NONE',  ( 199.0198855237646569, 7.818582849054650730, 18.41067656382650597 ) ) ;
#20041=CARTESIAN_POINT ( 'NONE',  ( -192.9588430854690273, 38.51493924976913519, 18.05360324515490333 ) ) ;
#20055=CARTESIAN_POINT ( 'NONE',  ( 200.0000000000000853, -18.97025941512468705, -1.247367644282773691 ) ) ;
#20060=CARTESIAN_POINT ( 'NONE',  ( 199.0179304339989415, -16.54579169021749863, -11.23843401478282544 ) ) ;
#20088=CARTESIAN_POINT ( 'NONE',  ( 200.0000000000000284, 7.828075510571024687, 17.32306842307162142 ) ) ;
#20094=CARTESIAN_POINT ( 'NONE',  ( -56.48582580120559271, 21.81201906317798489, -21.81201906317746619 ) ) ;
#20095=CARTESIAN_POINT ( 'NONE',  ( 199.0241407150285227, -2.291925048877014870, 19.87495682421008425 ) ) ;
#20120=CARTESIAN_POINT ( 'NONE',  ( 199.9999999999999432, 12.51862865053690577, 14.30364628684430706 ) ) ;
#20126=CARTESIAN_POINT ( 'NONE',  ( 199.0076473327615645, 2.278485796641462446, -19.86629856447459375 ) ) ;
#20134=CARTESIAN_POINT ( 'NONE',  ( 199.0164010208656009, 13.53619804287660777, 14.72436343555392035 ) ) ;
#20158=CARTESIAN_POINT ( 'NONE',  ( 200.0000000000001421, 16.91347576093571803, -8.662591770200990027 ) ) ;
#20159=CARTESIAN_POINT ( 'NONE',  ( 199.9999999999999432, -15.45674197124598592, 11.06829513483084426 ) ) ;
#20168=CARTESIAN_POINT ( 'NONE',  ( 199.0199585884774649, 7.679342959448028694, 18.46907803347260213 ) ) ;
#20169=CARTESIAN_POINT ( 'NONE',  ( 4.995406935893297984, 10.78321810390233892, -67.35176059882522281 ) ) ;
#20182=CARTESIAN_POINT ( 'NONE',  ( 199.9999999999996589, -18.97053056118941328, 1.250588282361275283 ) ) ;
#20184=( GEOMETRIC_REPRESENTATION_CONTEXT ( 3 ) GLOBAL_UNCERTAINTY_ASSIGNED_CONTEXT ( ( #19213 ) ) GLOBAL_UNIT_ASSIGNED_CONTEXT ( ( #10268, #14387, #2695 ) ) REPRESENTATION_CONTEXT ( 'NONE', 'WORKASPACE' ) );
#20186=CARTESIAN_POINT ( 'NONE',  ( 199.0200497209392267, -18.54142962866078648, -7.504851164020625021 ) ) ;
#20218=CARTESIAN_POINT ( 'NONE',  ( 199.9999999999999716, 8.673909288817675645, 16.91296503504769078 ) ) ;
#20226=CARTESIAN_POINT ( 'NONE',  ( 146.6084372240433709, -24.48358557860284179, -32.08495691632087699 ) ) ;
#20227=CARTESIAN_POINT ( 'NONE',  ( 199.0214920807345322, 4.534629261753806873, 19.48466678343157454 ) ) ;
#20253=CARTESIAN_POINT ( 'NONE',  ( 199.9999999999999716, 17.67195306284541090, 6.994325408928051324 ) ) ;
#20261=CARTESIAN_POINT ( 'NONE',  ( 199.0058919196228260, 8.838798596736017643, -17.93603902042922726 ) ) ;
#20266=CARTESIAN_POINT ( 'NONE',  ( 200.0000000000000853, -18.00470042792477798, 6.107801588486966082 ) ) ;
#20269=CARTESIAN_POINT ( 'NONE',  ( 199.0219179450577371, 3.573952992290374109, 19.68174087806957573 ) ) ;
#20295=CARTESIAN_POINT ( 'NONE',  ( 200.0000000000001137, 17.30391983412833667, 7.856783789979721710 ) ) ;
#20297=CARTESIAN_POINT ( 'NONE',  ( 199.9999999999999147, -12.54514294966348409, -14.28960723841028546 ) ) ;
#20306=CARTESIAN_POINT ( 'NONE',  ( 199.0213085020154153, 4.963412175948412219, 19.42123122998796703 ) ) ;
#20308=CARTESIAN_POINT ( 'NONE',  ( 170.2234770963711128, 10.92277846919216522, -10.92277846919186501 ) ) ;
#20310=CARTESIAN_POINT ( 'NONE',  ( 57.59792236341147031, 26.56190807104652052, 30.00663442387728708 ) ) ;
#20323=CARTESIAN_POINT ( 'NONE',  ( 199.0120775374408311, -7.960707704260069129, -18.34818886981279462 ) ) ;
#20352=CARTESIAN_POINT ( 'NONE',  ( 199.9999999999999716, 16.82276630623001878, 8.840806072347076494 ) ) ;
#20359=CARTESIAN_POINT ( 'NONE',  ( 192.4448373802100889, 14.14213562370330379, -14.14213562370292365 ) ) ;
#20360=CARTESIAN_POINT ( 'NONE',  ( 199.0235930299571123, -0.6679962965002699260, 20.00321896753086648 ) ) ;
#20385=ORIENTED_EDGE ( 'NONE', *, *, #13513, .F. ) ;
#20387=CARTESIAN_POINT ( 'NONE',  ( 199.9999999999999147, 11.56246421534694413, 15.09700933887624963 ) ) ;
#20395=CARTESIAN_POINT ( 'NONE',  ( 199.0104473268430922, -4.709499629590884417, -19.43548647772360383 ) ) ;
#20402=CARTESIAN_POINT ( 'NONE',  ( 199.9999999999999432, -13.87586802671829211, 12.99819774096606118 ) ) ;
#20405=CARTESIAN_POINT ( 'NONE',  ( 199.0238195103507053, -1.318470765087343954, 19.97100952642404437 ) ) ;
#20427=CARTESIAN_POINT ( 'NONE',  ( 199.9999999999998863, 18.47321080301961160, -4.449129010553737551 ) ) ;
#20428=CARTESIAN_POINT ( 'NONE',  ( 199.9999999999999716, -18.93198117488135779, -1.711693323776216191 ) ) ;
#20438=CARTESIAN_POINT ( 'NONE',  ( 199.0159431193063710, 14.16346371809618709, 14.12086452993616525 ) ) ;
#20439=CARTESIAN_POINT ( 'NONE',  ( -135.8532207217289738, -6.472252184283586729, -50.09629031063973770 ) ) ;
#20442=CARTESIAN_POINT ( 'NONE',  ( 163.1118516004056573, 9.006482792073693844, 47.56205970284970164 ) ) ;
#20457=CARTESIAN_POINT ( 'NONE',  ( 199.0171635947087907, -15.67013318013508716, -12.42972081464992407 ) ) ;
#20483=CARTESIAN_POINT ( 'NONE',  ( 199.9999999999998863, 15.61930985130600291, 10.83040361559445230 ) ) ;
#20491=CARTESIAN_POINT ( 'NONE',  ( -280.0000000000000000, -14.14213562373118549, 14.14213562373078936 ) ) ;
#20492=CARTESIAN_POINT ( 'NONE',  ( 199.0260264921024316, -10.00558763687667962, 17.32375098348098419 ) ) ;
#20506=CARTESIAN_POINT ( 'NONE',  ( -192.9588430854689989, 10.23066800230756712, -10.23066800230735396 ) ) ;
#20516=CARTESIAN_POINT ( 'NONE',  ( 199.9999999999999716, 17.24217208250532352, 8.000691389023806721 ) ) ;
#20522=CARTESIAN_POINT ( 'NONE',  ( 199.0139917666041924, -11.25641580849352685, -16.53121693397544689 ) ) ;
#20532=CARTESIAN_POINT ( 'NONE',  ( 199.0168302869249999, 12.92424399662411005, 15.26720349029574564 ) ) ;
#20560=CARTESIAN_POINT ( 'NONE',  ( 199.9999999999998579, 15.71915069317562264, -10.67410001769982308 ) ) ;
#20561=CARTESIAN_POINT ( 'NONE',  ( 199.9999999999999147, 10.80962424009062239, -15.62854876372556490 ) ) ;
#20570=CARTESIAN_POINT ( 'NONE',  ( 199.0157676419877646, 14.39733183096338998, 13.88287279058362067 ) ) ;
#20572=CARTESIAN_POINT ( 'NONE',  ( -105.3755690713226585, -15.38646221621738164, -41.18208027870615240 ) ) ;
#20574=CARTESIAN_POINT ( 'NONE',  ( -208.1127848780264742, 38.89260858015707356, 17.67593391476696141 ) ) ;
#20585=CARTESIAN_POINT ( 'NONE',  ( 199.0083412756643497, 0.3136196654984919618, -19.99640146592421175 ) ) ;
#20613=CARTESIAN_POINT ( 'NONE',  ( 200.0000000000000284, 15.35911892145054303, -11.18589804280325772 ) ) ;
#20618=CARTESIAN_POINT ( 'NONE',  ( 4.995406935893289102, 10.78321810389013002, -10.78321810388986712 ) ) ;
#20619=CARTESIAN_POINT ( 'NONE',  ( 199.0249556294982938, -5.033924301686514724, 19.36137939705603017 ) ) ;
#20654=CARTESIAN_POINT ( 'NONE',  ( 199.0257179982615128, -18.22226585379655361, 8.261159732268383848 ) ) ;
#20668=CARTESIAN_POINT ( 'NONE',  ( 199.0075440639197666, 19.83040477280651714, -2.587228267588620234 ) ) ;
#20675=CARTESIAN_POINT ( 'NONE',  ( -280.0000000000000000, -5.143516556418885058E-14, -6.902532920683853297E-30 ) ) ;
#20682=CARTESIAN_POINT ( 'NONE',  ( 199.0084359913980165, 0.06319087311583088118, -19.99616937079735379 ) ) ;
#20696=CARTESIAN_POINT ( 'NONE',  ( 199.9999999999998010, 4.312122466882670757, -18.50761716938983525 ) ) ;
#20699=CARTESIAN_POINT ( 'NONE',  ( 199.9999999999999147, 11.56007540354647389, -15.08186119327485386 ) ) ;
#20708=CARTESIAN_POINT ( 'NONE',  ( 199.0067131358059953, 19.32749934108755241, -5.289875845814065336 ) ) ;
#20709=CARTESIAN_POINT ( 'NONE',  ( 14.38125909742181285, -17.55144818341421598, -39.01709431150935359 ) ) ;
#20711=CARTESIAN_POINT ( 'NONE',  ( -86.96347745069644475, 41.18208027870576871, 15.38646221621837107 ) ) ;
#20725=CARTESIAN_POINT ( 'NONE',  ( 199.0247296274817188, -19.55681251529712128, 4.220088366773818045 ) ) ;
#20753=CARTESIAN_POINT ( 'NONE',  ( 199.9999999999998863, 18.97179924413623908, -1.226483293096950700 ) ) ;
#20756=CARTESIAN_POINT ( 'NONE',  ( 163.1118516004056573, -47.56205970284945295, -9.006482792074823607 ) ) ;
#20757=CARTESIAN_POINT ( 'NONE',  ( 199.0152755141893692, 15.03153897770602221, 13.19647528785794677 ) ) ;
#20783=CARTESIAN_POINT ( 'NONE',  ( 199.9999999999999716, -8.687076164477627316, 16.91209170048031041 ) ) ;
#20790=CARTESIAN_POINT ( 'NONE',  ( 199.0232268534825835, -20.00153578626446915, -0.3291254421221458948 ) ) ;
#20803=CARTESIAN_POINT ( 'NONE',  ( 199.0054597862206549, 11.64633275074771035, -16.26583636099561403 ) ) ;
#20818=CARTESIAN_POINT ( 'NONE',  ( 199.0153906436953264, -13.35702860092365363, -14.88696670886333706 ) ) ;
#20820=VERTEX_POINT ( 'NONE', #9790 ) ;
#20828=CARTESIAN_POINT ( 'NONE',  ( 199.9999999999999147, 0.2978356717867484682, -19.00168788844713319 ) ) ;
#20838=CARTESIAN_POINT ( 'NONE',  ( 199.0119115731982333, 18.47776054338839202, 7.648009306434410348 ) ) ;
#20839=CARTESIAN_POINT ( 'NONE',  ( -208.1127848780265026, 10.60833733269551615, -10.60833733269529766 ) ) ;
#20853=CARTESIAN_POINT ( 'NONE',  ( 199.0249934254769926, -19.32713910159323589, 5.171593721336591010 ) ) ;
#20885=CARTESIAN_POINT ( 'NONE',  ( 200.0000000000001990, 8.399020763088516972, -17.04381686846133803 ) ) ;
#20888=CARTESIAN_POINT ( 'NONE',  ( -56.48582580120559271, -6.472252184284276844, 6.472252184284108978 ) ) ;
#20889=CARTESIAN_POINT ( 'NONE',  ( 199.0124915487878923, 17.99959093953023270, 8.716253503037693307 ) ) ;
#20922=B_SPLINE_SURFACE_WITH_KNOTS ( 'NONE', 1, 3, ( 
 ( #18767, #16763, #24897, #21165, #22897, #4676, #6389, #14505, #22636, #8519, #2408, #16637, #10518, #24766, #14630, #22767, #9052, #23290, #3067, #5066, #25291, #13172, #21293, #19159, #7048, #15165, #943, #17157, #26004, #2048, #8015, #26277, #39, #15998, #24532, #22001, #7739, #20405, #12147, #16130, #22134, #10155, #18258, #10017, #8152, #14140, #24125, #14406, #24260, #20269, #1912, #6288, #13868, #2179, #10287, #15851, #3771, #11875, #2303, #5896, #22536, #6034, #19995, #12278, #6161, #22272, #18395, #16266, #172, #14004, #23981, #8278, #3915, #20532, #12014, #20134, #18125, #4046, #1781, #24395, #9885, #14271, #22407, #4183, #16404, #12407, #4317, #17853, #5760, #7877, #17986, #26134, #23192, #14798, #6683, #24934, #10689, #16797, #447, #14932, #4840, #25197, #4710, #18933, #22929, #24663, #581, #20937, #12534, #8413, #2715, #23069, #4440, #25064, #8551, #311, #12814, #18660, #20668, #10820, #16667, #14538, #10549, #18801, #22800, #715, #8819, #2437, #4577, #14660, #16535, #24798, #12674, #2848, #8688, #21195, #16930, #6816, #10412, #13080, #6550, #4972, #6944, #12946, #21062, #22668, #10956, #19062, #8954, #18530, #844, #17063, #6420, #15062, #20803, #2575, #6151, #22126, #2169, #19986, #18517, #20261, #3906, #18385, #8270, #2293, #8142, #22400, #31, #1770, #4038, #24386, #15987, #11866, #14261, #165, #7867, #10278, #12004, #3761, #2040, #20126, #24115, #16258, #1905, #17979, #13995, #22261, #26268, #4175, #12269, #5887, #8004, #18117, #9876, #10009, #16121, #6281, #14132, #24652, #20395, #16391, #13857, #16524, #24251, #298, #10403, #10143, #24523, #26125, #12137, #14396, #12397, #21992, #22528, #4308, #6025, #20522, #18247, #8402, #18789, #2834, #16784, #19051, #4829, #10943, #13066, #10538, #14525, #8942, #701, #4696, #10676, #16919, #6804, #24920, #25053, #2704, #12663, #2956, #14787, #8807, #6672, #21183, #2428, #17048, #25184, #22656, #18650, #435, #17175, #4567, #11066, #20925, #8539, #833, #21050, #22917, #6933, #14916, #15051, #20790, #4430, #23180, #2561, #9068, #570, #8675, #12798, #10809, #16656, #12934, #24787, #18919, #4959, #23057, #19179, #963, #6408, #12523, #20654, #22788, #6539, #14649, #11688, #3331, #21557, #13434, #25565, #5207, #19429, #5324, #21311, #23677, #3086, #11431, #5457, #3202 ),
 ( #3459, #19552, #9193, #25819, #7187, #19678, #1339, #15678, #17677, #13691, #1215, #7565, #23803, #21430, #5584, #21685, #25438, #17306, #11185, #11311, #9445, #1600, #17550, #25688, #13190, #11557, #7436, #21813, #15550, #15303, #9702, #9568, #25308, #7068, #13559, #13311, #1467, #3585, #19301, #9318, #17425, #7312, #15183, #15426, #23430, #23553, #19813, #23308, #5085, #1084, #16218, #14357, #11963, #24211, #3860, #22088, #7963, #12096, #5982, #18076, #20088, #1867, #8231, #20218, #10103, #26088, #6113, #23933, #22486, #16082, #1729, #1996, #12354, #4135, #9970, #12228, #15115, #17808, #26228, #14090, #22221, #3997, #25954, #18205, #8099, #24349, #14221, #15940, #20483, #16349, #17942, #6244, #22357, #20352, #5848, #2128, #4266, #10236, #2258, #18346, #127, #7696, #24481, #15808, #5710, #13814, #21948, #3724, #11827, #19945, #9837, #7823, #24072, #13954, #18748, #12760, #20753, #25147, #6367, #12896, #2793, #256, #14486, #22618, #21148, #8501, #15015, #24878, #4394, #4794, #25014, #529, #21010, #10768, #10905, #16614, #8365, #19017, #24747, #13028, #14613, #6502, #4527, #16745, #12488, #8768, #20613, #22879, #16883, #22748, #12625, #4916, #2523, #14748, #10640, #396, #796, #8899, #23145, #4656, #6634, #20885, #8635, #2663, #18881, #14880, #17010, #6898, #660, #6767, #23019, #24613, #10365, #18476, #2388, #16488, #10500, #18613, #23273, #17518, #1051, #19141, #9284, #11154, #13155, #15397, #19269, #7024, #3047, #11278, #15270, #11395, #3301, #5048, #23400, #7154, #925, #21275, #5176, #21650, #3174, #13656, #21525, #19517, #2922, #5548, #9157, #15643, #25784, #17392, #23645, #15143, #19399, #25657, #1434, #11031, #11524, #7403, #9035, #23521, #21401, #19649, #13279, #15515, #1182, #5423, #1304, #13526, #9533, #17268, #17139, #3422, #5293, #25532, #7280, #13401, #9412, #17643, #7534, #25403, #23770, #25274, #93, #11930, #5677, #5950, #16319, #8066, #13920, #16186, #3966, #21780, #22055, #9935, #24039, #3829, #3553, #14060, #20055, #1834, #12065, #19915, #24443, #12198, #21916, #10205, #15907, #20182, #9804, #7791, #8201, #5816, #6212, #1966, #10072, #11654, #24319, #26195, #18041, #19779, #18176, #6084, #18311, #14189, #17775, #1566, #26324, #2096, #7933, #9671, #25918, #22323, #16049, #7662, #24174, #15773, #22191, #4098 ) ),
 .UNSPECIFIED., .F., .T., .F.,
 ( 2, 2 ),
 ( 4, 2, 2, 2, 2, 2, 2, 2, 2, 2, 2, 2, 2, 2, 2, 2, 2, 2, 2, 2, 2, 2, 2, 2, 2, 2, 2, 2, 2, 2, 2, 2, 2, 2, 2, 2, 2, 2, 2, 2, 2, 2, 2, 2, 2, 2, 2, 2, 2, 2, 2, 2, 2, 2, 2, 2, 2, 2, 2, 2, 2, 2, 2, 2, 2, 2, 2, 2, 2, 2, 2, 2, 2, 2, 2, 2, 2, 2, 2, 2, 2, 2, 2, 2, 2, 2, 2, 2, 2, 2, 2, 2, 2, 2, 2, 2, 2, 2, 2, 2, 2, 2, 2, 2, 2, 2, 2, 2, 2, 2, 2, 2, 2, 2, 2, 2, 2, 2, 2, 2, 2, 2, 2, 2, 2, 2, 2, 2, 2, 2, 2, 2, 2, 2, 2, 2, 2, 2, 2, 2, 2, 2, 2, 2, 2, 2, 2, 2, 4 ),
 ( 0.000000000000000000, 1.000000000000000000 ),
 ( 0.001986339241202381145, 0.003842975313193646575, 0.004771293349189279290, 0.005235452367187095647, 0.005699611385184912005, 0.006163770403182728362, 0.006627929421180544720, 0.007092088439178361077, 0.007556247457176177434, 0.008484565493171810149, 0.009412883529167442864, 0.01034120156516307558, 0.01126951960115870829, 0.01173367861915652552, 0.01219783763715434101, 0.01266199665515215650, 0.01312615567314997372, 0.01405447370914560644, 0.01498279174514123915, 0.01683942781713250458, 0.01776774585312813903, 0.01869606388912377001, 0.01916022290712158377, 0.01962438192511940099, 0.02008854094311721822, 0.02055269996111503544, 0.02148101799711066989, 0.02240933603310630087, 0.02333765406910193185, 0.02426597210509756630, 0.02519429014109320075, 0.02565844915909101798, 0.02612260817708883173, 0.02658676719508664549, 0.02705092621308446271, 0.02797924424908009716, 0.02983588032107136259, 0.03076419835706699357, 0.03122835737506481080, 0.03169251639306262802, 0.03215667541106044525, 0.03262083442905826247, 0.03354915246505389692, 0.03447747050104953137, 0.03540578853704515888, 0.03633410657304078639, 0.03726242460903642084, 0.03772658362703423807, 0.03819074264503205529, 0.03865490166302987252, 0.03911906068102768974, 0.04004737871702332419, 0.04097569675301895864, 0.04283233282501022060, 0.04376065086100584811, 0.04468896889700148256, 0.04561728693299711701, 0.04654560496899275146, 0.04840224104098402036, 0.04933055907697965481, 0.05025887711297528232, 0.05072303613097309261, 0.05118719514897090983, 0.05165135416696872706, 0.05211551318496654428, 0.05304383122096217873, 0.05397214925695781318, 0.05490046729295344763, 0.05582878532894908208, 0.05675710336494471653, 0.05722126238294253375, 0.05768542140094034404, 0.05814958041893815432, 0.05861373943693597155, 0.05954205747293160600, 0.06139869354492287490, 0.06325532961691412992, 0.06511196568890539882, 0.06604028372490103327, 0.06696860176089666772, 0.06743276077889448494, 0.06789691979689230217, 0.06836107881489011939, 0.06882523783288793662, 0.06975355586888357107, 0.07068187390487920552, 0.07161019194087483997, 0.07253850997687047442, 0.07300266899486829164, 0.07346682801286610887, 0.07393098703086392609, 0.07439514604886174332, 0.07485930506685956054, 0.07532346408485737776, 0.07625178212085299834, 0.07810841819284425336, 0.07903673622883988781, 0.07950089524683770503, 0.07996505426483552226, 0.08042921328283333948, 0.08089337230083115671, 0.08182169033682679116, 0.08275000837282242561, 0.08367832640881806006, 0.08460664444481369451, 0.08553496248080932896, 0.08646328051680496340, 0.08692743953480278063, 0.08739159855280059785, 0.08785575757079841508, 0.08831991658879623230, 0.08924823462479186675, 0.09110487069678312178, 0.09203318873277874235, 0.09296150676877437680, 0.09342566578677219402, 0.09388982480477001125, 0.09435398382276782847, 0.09481814284076564570, 0.09574646087676128015, 0.09667477891275691460, 0.09760309694875254904, 0.09853141498474818349, 0.09899557400274600072, 0.09945973302074381794, 0.09992389203874163517, 0.1003880510567394524, 0.1022446871287307213, 0.1041013232007219902, 0.1050296412367176246, 0.1054938002547154419, 0.1059579592727132452, 0.1064221182907110486, 0.1068862773087088658, 0.1078145953447045002, 0.1096712314166957691, 0.1105995494526914036, 0.1115278674886870380, 0.1124561855246826725, 0.1133845035606783069, 0.1143128215966739414, 0.1152411396326695758, 0.1170977757046608447, 0.1180260937406564792, 0.1184902527586542964, 0.1189544117766521136, 0.1194185707946499309, 0.1198827298126477481, 0.1208110478486433687 ),
 .UNSPECIFIED. ) ;
#20925=CARTESIAN_POINT ( 'NONE',  ( 199.0212029771548430, -19.33411866963394488, -5.169619751639646488 ) ) ;
#20937=CARTESIAN_POINT ( 'NONE',  ( 199.0099419815959436, 19.67222971740176618, 3.604179563970075773 ) ) ;
#20959=CARTESIAN_POINT ( 'NONE',  ( 200.0000000000005116, -0.6320235832414241584, -19.00127953747481868 ) ) ;
#20960=CARTESIAN_POINT ( 'NONE',  ( 199.9999999999999147, -2.484827300297501207, -18.84147750260992638 ) ) ;
#20971=CARTESIAN_POINT ( 'NONE',  ( -208.1127848780264742, -17.67593391476605547, -38.89260858015755673 ) ) ;
#20985=CARTESIAN_POINT ( 'NONE',  ( 199.0205961407162931, -18.94296041394271768, -6.425165802706580997 ) ) ;
#21010=CARTESIAN_POINT ( 'NONE',  ( 199.9999999999998579, 17.67836847945686429, -6.970492097432807732 ) ) ;
#21014=CARTESIAN_POINT ( 'NONE',  ( 57.59792236341147031, -30.00663442387662627, -26.56190807104723461 ) ) ;
#21015=CARTESIAN_POINT ( 'NONE',  ( 199.0132385929227610, 17.30986399168244461, 10.02103235953326710 ) ) ;
#21035=ORIENTED_EDGE ( 'NONE', *, *, #9941, .F. ) ;
#21050=CARTESIAN_POINT ( 'NONE',  ( 199.0223302282441296, -19.84245377806801613, -2.613091800807908260 ) ) ;
#21058=AXIS2_PLACEMENT_3D ( 'NONE', #7994, #22, #15977 ) ;
#21062=CARTESIAN_POINT ( 'NONE',  ( 199.0054956575951621, 16.44889389956343706, -11.36889162147346255 ) ) ;
#21079=CARTESIAN_POINT ( 'NONE',  ( 199.0084075218435657, 0.1388852900563516679, -19.99583393261218589 ) ) ;
#21084=EDGE_LOOP ( 'NONE', ( #23710, #21035, #10806, #11338 ) ) ;
#21092=CARTESIAN_POINT ( 'NONE',  ( 199.9999999999998863, -4.016713260438497635, -18.57371263647062420 ) ) ;
#21095=CARTESIAN_POINT ( 'NONE',  ( 199.9999999999999147, -3.405556461844650329, -18.69721604853318908 ) ) ;
#21103=CARTESIAN_POINT ( 'NONE',  ( 199.0121267835791627, 18.30962774096152046, 8.053342476213535051 ) ) ;
#21104=CARTESIAN_POINT ( 'NONE',  ( 57.59792236341147031, -1.722363176415055985, 1.722363176415024677 ) ) ;
#21121=CARTESIAN_POINT ( 'NONE',  ( 200.0000000000000853, -13.44239485489230290, 13.44239485489200803 ) ) ;
#21148=CARTESIAN_POINT ( 'NONE',  ( 199.9999999999998863, 18.47321080301961160, -4.449129010553737551 ) ) ;
#21152=CARTESIAN_POINT ( 'NONE',  ( 199.0207542291320522, 6.104323864361830942, 19.05092312409432154 ) ) ;
#21165=CARTESIAN_POINT ( 'NONE',  ( 199.0263115711520072, -12.44642065545630238, 15.66510279686564289 ) ) ;
#21167=CARTESIAN_POINT ( 'NONE',  ( -91.56559293963834989, 12.25131212657428748, 44.31723036834913643 ) ) ;
#21178=CARTESIAN_POINT ( 'NONE',  ( 199.9999999999999147, 0.2942279655520377291, 19.00909807434749865 ) ) ;
#21183=CARTESIAN_POINT ( 'NONE',  ( 199.0196534518890701, -18.22073438007316071, -8.257363271777977687 ) ) ;
#21195=CARTESIAN_POINT ( 'NONE',  ( 199.0058938177734547, 17.94521767341456098, -8.824629201450257199 ) ) ;
#21213=CARTESIAN_POINT ( 'NONE',  ( 199.0118400166160200, -7.512756401568218223, -18.53321931831850478 ) ) ;
#21225=CARTESIAN_POINT ( 'NONE',  ( 200.0000000000001421, -10.69674284809226350, -15.70882504007707681 ) ) ;
#21235=CARTESIAN_POINT ( 'NONE',  ( 192.4448373802101173, -42.42640687122053578, -14.14213562370360577 ) ) ;
#21249=CARTESIAN_POINT ( 'NONE',  ( 199.0252366630825520, -19.04991887513223503, 6.114737037930856545 ) ) ;
#21275=CARTESIAN_POINT ( 'NONE',  ( 199.9999999999998863, -3.863658434880562265, -18.60611098383053630 ) ) ;
#21279=CARTESIAN_POINT ( 'NONE',  ( 199.0176798082135008, 11.64390658120213828, 16.27508030683247497 ) ) ;
#21293=CARTESIAN_POINT ( 'NONE',  ( 199.0254609980498799, -7.058152949095585882, 18.72097443096651403 ) ) ;
#21295=CARTESIAN_POINT ( 'NONE',  ( -259.2033419157646676, 21.55415060305790931, 35.01439189186571355 ) ) ;
#21301=CARTESIAN_POINT ( 'NONE',  ( 4.995406935893289102, 10.78321810389013002, -10.78321810388986712 ) ) ;
#21311=CARTESIAN_POINT ( 'NONE',  ( 199.0263429660336385, -15.25543418246514982, 12.94225785457335753 ) ) ;
#21315=CIRCLE ( 'NONE', #24289, 10.00000000000000000 ) ;
#21338=VERTEX_POINT ( 'NONE', #17307 ) ;
#21340=CARTESIAN_POINT ( 'NONE',  ( 199.0206683190968135, -19.03253901574858986, -6.320310628391184515 ) ) ;
#21343=VERTEX_POINT ( 'NONE', #1468 ) ;
#21353=CARTESIAN_POINT ( 'NONE',  ( 200.0000000000001421, -12.54320094651582451, -14.29122475987005458 ) ) ;
#21378=CARTESIAN_POINT ( 'NONE',  ( 200.0000000000001421, -0.6349535514222880428, 19.00853270881595591 ) ) ;
#21401=CARTESIAN_POINT ( 'NONE',  ( 199.9999999999998863, -11.20618975336454071, -15.34975362513495689 ) ) ;
#21404=CARTESIAN_POINT ( 'NONE',  ( 199.0071786209885261, 3.739031945787267386, -19.64359944086908527 ) ) ;
#21425=ORIENTED_EDGE ( 'NONE', *, *, #6153, .T. ) ;
#21430=CARTESIAN_POINT ( 'NONE',  ( 199.9999999999998863, -9.643221244315762775, 16.38360543750208009 ) ) ;
#21437=CYLINDRICAL_SURFACE ( 'NONE', #5471, 10.00000000000000000 ) ;
#21458=ORIENTED_EDGE ( 'NONE', *, *, #16287, .T. ) ;
#21460=CARTESIAN_POINT ( 'NONE',  ( 199.0255849842728253, -18.49502280213427952, 7.623850636981702955 ) ) ;
#21468=CARTESIAN_POINT ( 'NONE',  ( 199.9999999999999147, -13.65919145721374761, -13.21838778087559518 ) ) ;
#21482=CARTESIAN_POINT ( 'NONE',  ( 170.2234770963711128, -17.36149277827010096, 17.36149277826970660 ) ) ;
#21503=CARTESIAN_POINT ( 'NONE',  ( 199.9999999999998863, 8.393744152662998559, 17.05383455604227905 ) ) ;
#21525=CARTESIAN_POINT ( 'NONE',  ( 199.9999999999998863, -5.231270638550959085, -18.27112563740264761 ) ) ;
#21529=CARTESIAN_POINT ( 'NONE',  ( 199.0058919196228260, 8.838798596736017643, -17.93603902042922726 ) ) ;
#21548=CARTESIAN_POINT ( 'NONE',  ( -135.8532207217289738, -6.472252184284280396, 6.472252184284099208 ) ) ;
#21557=CARTESIAN_POINT ( 'NONE',  ( 199.0262399469797572, -16.26902294624164469, 11.64593733880351500 ) ) ;
#21587=CARTESIAN_POINT ( 'NONE',  ( 199.0168320490197402, -15.28088196978702129, -12.92611743443934813 ) ) ;
#21596=CARTESIAN_POINT ( 'NONE',  ( -280.0000000000000000, 14.14213562373108424, -14.14213562373078759 ) ) ;
#21598=CARTESIAN_POINT ( 'NONE',  ( 199.9999999999998295, -19.00894346483091724, 0.1575548292166454312 ) ) ;
#21623=CARTESIAN_POINT ( 'NONE',  ( 199.9999999999998863, 9.495902909754645904, 16.46521490772419583 ) ) ;
#21650=CARTESIAN_POINT ( 'NONE',  ( 199.9999999999998863, -4.322767242657778120, -18.50495320732392557 ) ) ;
#21654=CARTESIAN_POINT ( 'NONE',  ( 199.0068982850735608, 19.44025291972790370, -4.682182605709538592 ) ) ;
#21685=CARTESIAN_POINT ( 'NONE',  ( 199.9999999999998863, -9.236595569432955344, 16.61620204157069125 ) ) ;
#21699=DIRECTION ( 'NONE',  ( -1.000000000000000000, -1.836970198721030181E-16, -2.465190328815661892E-32 ) ) ;
#21714=CARTESIAN_POINT ( 'NONE',  ( 199.0260502585402378, -17.33706145817157562, 10.06788908951285499 ) ) ;
#21728=CARTESIAN_POINT ( 'NONE',  ( 199.9999999999996589, -18.97053056118941328, 1.250588282361275283 ) ) ;
#21754=CARTESIAN_POINT ( 'NONE',  ( 199.9999999999998863, 12.28125103214278901, 14.50804496155330447 ) ) ;
#21768=CARTESIAN_POINT ( 'NONE',  ( 91.82158438592158234, 16.11829626348378142, 40.45024623143977749 ) ) ;
#21780=CARTESIAN_POINT ( 'NONE',  ( 200.0000000000000000, -18.09920287623689106, -5.808051173427421610 ) ) ;
#21783=CARTESIAN_POINT ( 'NONE',  ( 199.0058364129993436, 9.132953877242854901, -17.78802470895853816 ) ) ;
#21801=CARTESIAN_POINT ( 'NONE',  ( 57.59792236341147031, -1.722363176415055985, 1.722363176415024677 ) ) ;
#21813=CARTESIAN_POINT ( 'NONE',  ( 199.9999999999996305, -4.934527571401590151, 18.35877764772902410 ) ) ;
#21819=CARTESIAN_POINT ( 'NONE',  ( -192.9588430854689989, 38.51493924976983152, -38.51493924976893624 ) ) ;
#21847=CARTESIAN_POINT ( 'NONE',  ( 199.0255387882960747, -18.58171137233306780, 7.410670782471526330 ) ) ;
#21856=CARTESIAN_POINT ( 'NONE',  ( 14.38125909742181108, 39.01709431150961649, -39.01709431150867147 ) ) ;
#21858=CARTESIAN_POINT ( 'NONE',  ( 199.9999999999999716, -14.18957598410689869, 12.65210747703644500 ) ) ;
#21885=CARTESIAN_POINT ( 'NONE',  ( 199.9999999999998863, -9.643221244315762775, 16.38360543750208009 ) ) ;
#21886=CARTESIAN_POINT ( 'NONE',  ( 199.9999999999998863, -18.28231079023461092, -5.210528357603022798 ) ) ;
#21898=CARTESIAN_POINT ( 'NONE',  ( 0.2972598230769886718, 38.42060263243643448, 18.14793986248763957 ) ) ;
#21916=CARTESIAN_POINT ( 'NONE',  ( 200.0000000000000000, -19.00702131438069031, 0.3144861700050793352 ) ) ;
#21921=CARTESIAN_POINT ( 'NONE',  ( 199.0070393743141892, 19.55016766319115007, -4.199986046643529924 ) ) ;
#21939=EDGE_LOOP ( 'NONE', ( #1333, #21458, #2119, #733 ) ) ;
#21948=CARTESIAN_POINT ( 'NONE',  ( 200.0000000000000853, 18.51119012207909620, 4.337730402235636440 ) ) ;
#21956=CARTESIAN_POINT ( 'NONE',  ( 200.0000000000000000, 42.42640687119267540, 14.14213562373153543 ) ) ;
#21984=CARTESIAN_POINT ( 'NONE',  ( 199.9999999999999147, 18.82040333305158342, 2.653950712460805494 ) ) ;
#21992=CARTESIAN_POINT ( 'NONE',  ( 199.0134806391063194, -10.42534412885540185, -17.06722571675988931 ) ) ;
#21998=CARTESIAN_POINT ( 'NONE',  ( 199.9999999999998579, -18.51658467707331113, 4.312655811444462195 ) ) ;
#22001=CARTESIAN_POINT ( 'NONE',  ( 199.0242446922718784, -2.616032970993653173, 19.83497009005848710 ) ) ;
#22020=EDGE_LOOP ( 'NONE', ( #7822, #255, #25206, #25144, #17293 ) ) ;
#22028=DIRECTION ( 'NONE',  ( 1.298934084353256076E-16, -0.7071067811865561215, 0.7071067811865389130 ) ) ;
#22029=CARTESIAN_POINT ( 'NONE',  ( 199.9999999999998863, 18.88157209772827017, -2.150785294275829429 ) ) ;
#22030=CARTESIAN_POINT ( 'NONE',  ( 200.0000000000000000, -15.45605508098274861, -11.06530458668214933 ) ) ;
#22041=CARTESIAN_POINT ( 'NONE',  ( 199.0231640206657460, 0.4968506554899906891, 19.99832409911510211 ) ) ;
#22043=CARTESIAN_POINT ( 'NONE',  ( -198.0356074513804572, 67.44298959250878056, -10.87444709758402261 ) ) ;
#22046=CARTESIAN_POINT ( 'NONE',  ( -135.8532207217289738, -6.472252184284280396, 6.472252184284099208 ) ) ;
#22055=CARTESIAN_POINT ( 'NONE',  ( 199.9999999999998863, -18.14641137086378819, -5.658975142792487922 ) ) ;
#22059=CARTESIAN_POINT ( 'NONE',  ( 199.0174211633917878, -15.97280307358279039, -12.03849830368706009 ) ) ;
#22078=PRODUCT_CONTEXT ( 'NONE', #2450, 'mechanical' ) ;
#22087=ORIENTED_EDGE ( 'NONE', *, *, #9807, .T. ) ;
#22088=CARTESIAN_POINT ( 'NONE',  ( 200.0000000000000000, 5.800536564436440834, 18.10358378745109320 ) ) ;
#22094=CARTESIAN_POINT ( 'NONE',  ( 163.1118516004056573, -19.27778845539181063, -37.29075403953176959 ) ) ;
#22120=CARTESIAN_POINT ( 'NONE',  ( 199.9999999999999432, 18.36080785346942434, 4.936233792941779441 ) ) ;
#22126=CARTESIAN_POINT ( 'NONE',  ( 199.0056860580130262, 9.997888132351027579, -17.31887563448481160 ) ) ;
#22131=CARTESIAN_POINT ( 'NONE',  ( 200.0000000000001421, -15.08701489606589341, 11.56722645162647467 ) ) ;
#22134=CARTESIAN_POINT ( 'NONE',  ( 199.0231121918538975, 0.6363371645724309467, 19.99606429142543362 ) ) ;
#22164=CARTESIAN_POINT ( 'NONE',  ( 200.0000000000002558, 17.05253901346626222, -8.385556056821480198 ) ) ;
#22167=CARTESIAN_POINT ( 'NONE',  ( 199.9999999999999432, -18.76513715205313559, -3.093437544788904869 ) ) ;
#22177=CARTESIAN_POINT ( 'NONE',  ( 199.0232603141898551, 0.2386269578223878252, 20.00239709541226674 ) ) ;
#22178=CARTESIAN_POINT ( 'NONE',  ( -259.2033419157646676, 21.55415060305860209, -21.55415060305812602 ) ) ;
#22180=CARTESIAN_POINT ( 'NONE',  ( -238.4067589809705794, 0.6820004457912851592, -0.6820004457913123597 ) ) ;
#22191=CARTESIAN_POINT ( 'NONE',  ( 199.9999999999999432, -13.66164182518334691, 13.22314710892283074 ) ) ;
#22194=CARTESIAN_POINT ( 'NONE',  ( 199.0108247880216368, -5.504876786518239307, -19.22761790364454271 ) ) ;
#22221=CARTESIAN_POINT ( 'NONE',  ( 199.9999999999996874, 13.64679526057751069, 13.22824625860694070 ) ) ;
#22227=CARTESIAN_POINT ( 'NONE',  ( -105.3755690713226585, -15.38646221621738164, -41.18208027870615240 ) ) ;
#22228=CARTESIAN_POINT ( 'NONE',  ( 199.0250816517838359, -5.508431349499541163, 19.23181920140171997 ) ) ;
#22254=CARTESIAN_POINT ( 'NONE',  ( 199.9999999999999716, 16.13598342540508668, 10.05825190933999203 ) ) ;
#22261=CARTESIAN_POINT ( 'NONE',  ( 199.0082207658673781, 0.6402583678929150146, -19.98857080023024579 ) ) ;
#22268=CARTESIAN_POINT ( 'NONE',  ( 199.9999999999998579, -17.68075590865577951, 6.990562776172230208 ) ) ;
#22272=CARTESIAN_POINT ( 'NONE',  ( 199.0189287881835583, 9.564175521352543896, 17.56735958655279362 ) ) ;
#22297=CARTESIAN_POINT ( 'NONE',  ( 200.0000000000001421, 17.31676413174603013, -7.825505819403215213 ) ) ;
#22298=CARTESIAN_POINT ( 'NONE',  ( 199.9999999999999432, -18.94552238787882104, -1.555198626918513849 ) ) ;
#22307=CARTESIAN_POINT ( 'NONE',  ( 199.0252590766962726, -6.209579518222142269, 19.01904426816868110 ) ) ;
#22309=CARTESIAN_POINT ( 'NONE',  ( 146.6084372240433709, 32.08495691632030145, 24.48358557860365181 ) ) ;
#22312=CARTESIAN_POINT ( 'NONE',  ( -91.56559293963834989, 40.53558337403654832, 16.03295912088756481 ) ) ;
#22323=CARTESIAN_POINT ( 'NONE',  ( 200.0000000000002274, -14.59760583945227808, 12.17906594671359244 ) ) ;
#22326=CARTESIAN_POINT ( 'NONE',  ( 199.0097193260481561, -3.097360908056462137, -19.75623422735097989 ) ) ;
#22357=CARTESIAN_POINT ( 'NONE',  ( 200.0000000000001421, 16.60215271479902910, 9.252637072649047667 ) ) ;
#22366=CARTESIAN_POINT ( 'NONE',  ( 136.1360204305621266, 3.511608612530757068, -3.511608612530642937 ) ) ;
#22367=CARTESIAN_POINT ( 'NONE',  ( 199.0224671581742371, 2.272106995489924230, 19.87442369886018767 ) ) ;
#22393=CARTESIAN_POINT ( 'NONE',  ( 199.9999999999999716, 14.28780111431841782, 12.54737623376984956 ) ) ;
#22400=CARTESIAN_POINT ( 'NONE',  ( 199.0062089136474128, 7.336486126005011599, -18.60345363517511430 ) ) ;
#22402=DIRECTION ( 'NONE',  ( -1.000000000000000000, -1.836970198721030181E-16, -2.465190328815661892E-32 ) ) ;
#22407=CARTESIAN_POINT ( 'NONE',  ( 199.0155347402294410, 14.70064717653387554, 13.56132639103557125 ) ) ;
#22433=CARTESIAN_POINT ( 'NONE',  ( 199.9999999999999716, 16.82276630623001878, 8.840806072347076494 ) ) ;
#22434=CARTESIAN_POINT ( 'NONE',  ( 199.9999999999999147, -18.52392551398779830, 4.314389638746997768 ) ) ;
#22444=CARTESIAN_POINT ( 'NONE',  ( -198.0356074513804572, 10.87444709761036066, -67.44298959253325165 ) ) ;
#22446=CARTESIAN_POINT ( 'NONE',  ( 130.8568914410475088, 32.49135343045448820, 24.07718906446946860 ) ) ;
#22459=CARTESIAN_POINT ( 'NONE',  ( 199.0173355507466226, -15.87315179554041045, -12.16952887920782445 ) ) ;
#22486=CARTESIAN_POINT ( 'NONE',  ( 200.0000000000000284, 9.630262036685882876, 16.38694142346205140 ) ) ;
#22493=CARTESIAN_POINT ( 'NONE',  ( -135.8532207217289738, -34.75652343174584757, -21.81201906317816253 ) ) ;
#22521=CARTESIAN_POINT ( 'NONE',  ( 199.9999999999999432, 6.682224494514668933, 17.80490695329945439 ) ) ;
#22528=CARTESIAN_POINT ( 'NONE',  ( 199.0135655005340425, -10.56572504866429973, -16.98073106299600710 ) ) ;
#22536=CARTESIAN_POINT ( 'NONE',  ( 199.0196638708318631, 8.237985373594881366, 18.22956011771260165 ) ) ;
#22561=CARTESIAN_POINT ( 'NONE',  ( 199.9999999999998863, 18.74710533595338546, 3.118879735276928855 ) ) ;
#22562=CARTESIAN_POINT ( 'NONE',  ( 199.9999999999999432, 3.553227108789564159, -18.66636905392490675 ) ) ;
#22565=FACE_OUTER_BOUND ( 'NONE', #14389, .T. ) ;
#22572=CARTESIAN_POINT ( 'NONE',  ( 199.0189648287746991, 9.496445123477679218, 17.61199005508735738 ) ) ;
#22573=CARTESIAN_POINT ( 'NONE',  ( 184.8905102610680444, 13.49065550809826952, -13.49065550809790359 ) ) ;
#22575=CARTESIAN_POINT ( 'NONE',  ( 170.2234770963711128, 39.20704971665372796, 17.36149277827039583 ) ) ;
#22591=CARTESIAN_POINT ( 'NONE',  ( 199.0145894657785846, -12.18649378798404470, -15.86093292504746621 ) ) ;
#22618=CARTESIAN_POINT ( 'NONE',  ( 199.9999999999998863, 18.50936851023984886, -4.296315843485498220 ) ) ;
#22624=CARTESIAN_POINT ( 'NONE',  ( -105.3755690713226727, -15.38646221621807619, 15.38646221621768362 ) ) ;
#22625=CARTESIAN_POINT ( 'NONE',  ( 199.0244464070843833, -3.263486543644114946, 19.73887645897787735 ) ) ;
#22636=CARTESIAN_POINT ( 'NONE',  ( 199.0261966595921592, -11.26051109717869458, 16.53566845662597729 ) ) ;
#22638=FACE_OUTER_BOUND ( 'NONE', #23967, .T. ) ;
#22656=CARTESIAN_POINT ( 'NONE',  ( 199.0202851408366485, -18.72068532052425383, -7.046142524300833543 ) ) ;
#22668=CARTESIAN_POINT ( 'NONE',  ( 199.0054653064281922, 16.25946365448332998, -11.63817148238572940 ) ) ;
#22681=CARTESIAN_POINT ( 'NONE',  ( 199.0138805921241953, -11.07098026833737414, -16.66790957460414901 ) ) ;
#22692=CARTESIAN_POINT ( 'NONE',  ( 199.9999999999999716, -5.826418053481885906, -18.09029720167993105 ) ) ;
#22701=CARTESIAN_POINT ( 'NONE',  ( 199.0082414334414125, 19.98886982631870524, -0.5857068698800287354 ) ) ;
#22702=CARTESIAN_POINT ( 'NONE',  ( 151.7948205124836250, 4.785054706301759886, -4.785054706301612448 ) ) ;
#22704=CARTESIAN_POINT ( 'NONE',  ( -56.48582580120559982, 21.81201906317729922, 34.75652343174635917 ) ) ;
#22716=CARTESIAN_POINT ( 'NONE',  ( 200.0000000000000568, -10.82911035642265141, 15.62521814345774196 ) ) ;
#22719=CARTESIAN_POINT ( 'NONE',  ( 199.9999999999998863, 13.43021917686961331, -13.43983678748323918 ) ) ;
#22740=ADVANCED_FACE ( 'NONE', ( #415 ), #20922, .T. ) ;
#22748=CARTESIAN_POINT ( 'NONE',  ( 199.9999999999998295, 14.29413690760092592, -12.53266873553815053 ) ) ;
#22752=CARTESIAN_POINT ( 'NONE',  ( -91.56559293963834989, -16.03295912088728414, 16.03295912088688269 ) ) ;
#22753=CARTESIAN_POINT ( 'NONE',  ( 199.0147602753770855, 15.66021538362855381, 12.44349737331557648 ) ) ;
#22767=CARTESIAN_POINT ( 'NONE',  ( 199.0259813356335883, -9.719824439858887999, 17.48565896982476175 ) ) ;
#22782=CARTESIAN_POINT ( 'NONE',  ( 199.9999999999999716, -7.851686492350575364, 17.31563863434756101 ) ) ;
#22788=CARTESIAN_POINT ( 'NONE',  ( 199.0258314272957421, -17.94308652430182605, 8.851303907023687856 ) ) ;
#22799=DIRECTION ( 'NONE',  ( 0.000000000000000000, -1.000000000000000000, 0.000000000000000000 ) ) ;
#22800=CARTESIAN_POINT ( 'NONE',  ( 199.0068982850735608, 19.44025291972790370, -4.682182605709538592 ) ) ;
#22814=CARTESIAN_POINT ( 'NONE',  ( 199.0116092925779014, -7.071658929006641614, -18.70726711289027833 ) ) ;
#22827=CARTESIAN_POINT ( 'NONE',  ( 200.0000000000001137, 2.164978928433492822, -18.87806096587463855 ) ) ;
#22840=CARTESIAN_POINT ( 'NONE',  ( 136.1360204305621551, -53.05693388239309627, -3.511608612531332163 ) ) ;
#22853=CARTESIAN_POINT ( 'NONE',  ( 199.0202851408366485, -18.72068532052425383, -7.046142524300833543 ) ) ;
#22879=CARTESIAN_POINT ( 'NONE',  ( 200.0000000000003126, 15.08009544811998204, -11.56244146370294779 ) ) ;
#22882=CARTESIAN_POINT ( 'NONE',  ( 163.1118516004056573, -19.27778845538787422, 19.27778845538743724 ) ) ;
#22883=CARTESIAN_POINT ( 'NONE',  ( 199.0142490642952566, 16.24935999037262846, 11.66321269349018941 ) ) ;
#22897=CARTESIAN_POINT ( 'NONE',  ( 199.0262910934941942, -12.18938195246538037, 15.86593956234834479 ) ) ;
#22899=CARTESIAN_POINT ( 'NONE',  ( -259.2033419157646676, -6.730120644403663199, 6.730120644403451813 ) ) ;
#22917=CARTESIAN_POINT ( 'NONE',  ( 199.0227232939661519, -19.93874224789216143, -1.638880401382246443 ) ) ;
#22929=CARTESIAN_POINT ( 'NONE',  ( 199.0111318983613842, 19.03723981379789265, 6.131360352008743853 ) ) ;
#22955=CARTESIAN_POINT ( 'NONE',  ( 199.9999999999999716, 14.88808753490056880, -11.80862348214050606 ) ) ;
#22966=CARTESIAN_POINT ( 'NONE',  ( 199.0110640845461489, 19.08185933734193895, 5.992088389419413019 ) ) ;
#22968=CARTESIAN_POINT ( 'NONE',  ( 57.59792236341147031, -30.00663442387662627, -26.56190807104723461 ) ) ;
#22987=CARTESIAN_POINT ( 'NONE',  ( 199.0248198352711313, -19.48551319141294869, 4.538181572781159190 ) ) ;
#23013=AXIS2_PLACEMENT_3D ( 'NONE', #1122, #2265, #10243 ) ;
#23019=CARTESIAN_POINT ( 'NONE',  ( 199.9999999999998010, 5.803429233430792422, -18.09525674440013177 ) ) ;
#23022=CARTESIAN_POINT ( 'NONE',  ( -91.56559293963834989, -44.31723036834885932, -12.25131212657538171 ) ) ;
#23023=CARTESIAN_POINT ( 'NONE',  ( 199.0075440639197666, 19.83040477280651714, -2.587228267588620234 ) ) ;
#23052=CARTESIAN_POINT ( 'NONE',  ( 199.9999999999999432, -13.00408651859840958, 13.88070474188551451 ) ) ;
#23057=CARTESIAN_POINT ( 'NONE',  ( 199.0252366630825520, -19.04991887513223503, 6.114737037930856545 ) ) ;
#23069=CARTESIAN_POINT ( 'NONE',  ( 199.0091071337781159, 19.93120984291649478, 1.649067560610785854 ) ) ;
#23096=CARTESIAN_POINT ( 'NONE',  ( 200.0000000000001705, 5.211075256460824257, -18.27473396828003871 ) ) ;
#23097=CARTESIAN_POINT ( 'NONE',  ( 199.9999999999999716, 3.398245514232853814, -18.69524394795535827 ) ) ;
#23105=CARTESIAN_POINT ( 'NONE',  ( 199.0123650023721495, 18.11534524532891766, 8.488184440863852487 ) ) ;
#23106=CARTESIAN_POINT ( 'NONE',  ( -213.1075012329537230, -18.58567234101102272, -37.98287015391260013 ) ) ;
#23119=CARTESIAN_POINT ( 'NONE',  ( 199.0263730241462099, -14.60190056250242030, 13.67829565473005715 ) ) ;
#23145=CARTESIAN_POINT ( 'NONE',  ( 199.9999999999998863, 9.229831349313808886, -16.61069465220444386 ) ) ;
#23149=CARTESIAN_POINT ( 'NONE',  ( 199.0145894300637792, 15.86095929198710586, 12.18642508278280623 ) ) ;
#23164=CARTESIAN_POINT ( 'NONE',  ( -30.26275506840325136, 29.48230279907760121, 27.08623969584625613 ) ) ;
#23176=CARTESIAN_POINT ( 'NONE',  ( 199.9999999999999716, -9.646513317630143192, 16.38616289770262568 ) ) ;
#23180=CARTESIAN_POINT ( 'NONE',  ( 199.0234090143162859, -20.00365258984362882, 0.1656111763342176801 ) ) ;
#23192=CARTESIAN_POINT ( 'NONE',  ( 199.0130717410369812, 17.47129959974107294, 9.736724163761770967 ) ) ;
#23208=CARTESIAN_POINT ( 'NONE',  ( 199.0075023815175825, 2.710256083316576081, -19.82277908217579920 ) ) ;
#23213=EDGE_LOOP ( 'NONE', ( #3105, #20385, #1502, #16847 ) ) ;
#23220=CARTESIAN_POINT ( 'NONE',  ( 200.0000000000002274, -18.85575486854367355, -2.482946933799725642 ) ) ;
#23230=CARTESIAN_POINT ( 'NONE',  ( 199.0061349475965358, 18.46602535085470009, -7.668765344048432908 ) ) ;
#23232=CARTESIAN_POINT ( 'NONE',  ( -162.0762913951021176, -27.08623940707584055, -29.48230308784799547 ) ) ;
#23248=CARTESIAN_POINT ( 'NONE',  ( 199.0262110011730954, -16.45735938206000171, 11.37817034370231006 ) ) ;
#23273=CARTESIAN_POINT ( 'NONE',  ( 200.0000000000000000, 2.939587388390868306, -18.77290383772223592 ) ) ;
#23277=CARTESIAN_POINT ( 'NONE',  ( 199.0089741461167989, 19.95552976068599804, 1.321036586804004820 ) ) ;
#23290=CARTESIAN_POINT ( 'NONE',  ( 199.0258842571097375, -9.142960865851959440, 17.79628948870135829 ) ) ;
#23292=CARTESIAN_POINT ( 'NONE',  ( -280.0000000000000568, 14.14213562373038968, 42.42640687119305198 ) ) ;
#23301=ORIENTED_EDGE ( 'NONE', *, *, #9941, .T. ) ;
#23308=CARTESIAN_POINT ( 'NONE',  ( 199.9999999999998579, 2.934899133129863280, 18.78102297366244500 ) ) ;
#23338=CARTESIAN_POINT ( 'NONE',  ( 199.0199226726568895, -18.44042569010415633, -7.747917312412542223 ) ) ;
#23349=CARTESIAN_POINT ( 'NONE',  ( 199.9999999999998863, -17.04947422730185025, -8.406841951002201441 ) ) ;
#23359=CARTESIAN_POINT ( 'NONE',  ( -30.26275506840324070, -27.08623969584554558, -29.48230279907826912 ) ) ;
#23369=( BOUNDED_SURFACE ( )  B_SPLINE_SURFACE ( 3, 3, ( 
 ( #3678, #3413, #22180, #13515, #19640, #9524, #1823, #5804, #22046, #18167, #7649, #5413, #15763, #26182, #8057, #5939, #5668, #13774, #11786, #1690, #16038, #18031, #23634, #19906, #25774, #9794, #7525, #15633, #23758, #5539 ),
 ( #13645, #17897, #26045, #7782, #20574, #2219, #12446, #24570, #14312, #8455, #2346, #18704, #10458, #22704, #8594, #351, #4480, #6075, #4088, #20310, #487, #12581, #24433, #212, #12188, #20442, #16704, #16574, #24836, #18571 ),
 ( #10328, #24705, #18437, #6459, #16173, #8321, #14177, #2087, #10589, #12315, #24308, #22312, #20711, #14575, #18297, #2477, #16309, #10194, #83, #8193, #6200, #22446, #4226, #16446, #6326, #14448, #22575, #4353, #19820, #21956 ),
 ( #4143, #133, #14098, #26095, #11695, #9709, #21819, #7969, #2134, #26235, #11970, #7831, #8237, #20094, #1873, #1606, #9844, #17814, #16355, #3730, #13960, #17948, #22366, #13696, #9976, #19951, #12235, #5717, #20359, #15949 ),
 ( #10242, #11833, #3868, #25960, #24080, #18353, #10110, #5590, #5989, #22227, #1943, #18084, #4003, #1735, #3590, #7703, #14227, #15814, #8105, #23940, #12102, #13822, #16088, #20226, #5854, #22094, #24218, #2004, #18211, #16226 ),
 ( #24355, #6119, #16620, #10643, #8372, #25017, #6373, #534, #22493, #8639, #8903, #23022, #19020, #6637, #18620, #4272, #2264, #14363, #16749, #21014, #18751, #4531, #403, #799, #12629, #20756, #12360, #2394, #10372, #24488 ),
 ( #20491, #8772, #10908, #18482, #263, #12899, #6250, #24881, #4660, #22624, #10506, #22752, #12493, #20888, #16494, #2796, #20618, #8506, #6771, #12763, #24619, #2526, #18885, #14491, #14751, #22882, #14883, #4399, #24753, #10772 ) ),
 .UNSPECIFIED., .T., .F., .F. ) 
 B_SPLINE_SURFACE_WITH_KNOTS ( ( 4, 3, 4 ),
 ( 4, 2, 2, 2, 2, 2, 2, 2, 2, 2, 2, 2, 2, 2, 4 ),
 ( 0.000000000000000000, 0.5000000000000000000, 1.000000000000000000 ),
 ( 0.000000000000000000, 0.1357259735107005372, 0.1651108541090157700, 0.1944957347073310028, 0.3598804999793158710, 0.3867117631979620773, 0.4135430264166082281, 0.5789277916885930964, 0.6062785021374117456, 0.6336292125862302838, 0.8508620842112317728, 0.8814014469398914198, 0.9119408096685510667, 0.9559704048342755334, 1.000000000000000000 ),
 .UNSPECIFIED. ) 
 GEOMETRIC_REPRESENTATION_ITEM ( )  RATIONAL_B_SPLINE_SURFACE ( (
 ( 1.000000000000000000, 1.000000000000000000, 1.000000000000000000, 1.000000000000000000, 1.000000000000000000, 1.000000000000000000, 1.000000000000000000, 1.000000000000000000, 1.000000000000000000, 1.000000000000000000, 1.000000000000000000, 1.000000000000000000, 1.000000000000000000, 1.000000000000000000, 1.000000000000000000, 1.000000000000000000, 1.000000000000000000, 1.000000000000000000, 1.000000000000000000, 1.000000000000000000, 1.000000000000000000, 1.000000000000000000, 1.000000000000000000, 1.000000000000000000, 1.000000000000000000, 1.000000000000000000, 1.000000000000000000, 1.000000000000000000, 1.000000000000000000, 1.000000000000000000),
 ( 0.3333333333333333703, 0.3333333333333333703, 0.3333333333333333703, 0.3333333333333333703, 0.3333333333333333703, 0.3333333333333333703, 0.3333333333333333703, 0.3333333333333333703, 0.3333333333333333703, 0.3333333333333333703, 0.3333333333333333703, 0.3333333333333333703, 0.3333333333333333703, 0.3333333333333333703, 0.3333333333333333703, 0.3333333333333333703, 0.3333333333333333703, 0.3333333333333333703, 0.3333333333333333703, 0.3333333333333333703, 0.3333333333333333703, 0.3333333333333333703, 0.3333333333333333703, 0.3333333333333333703, 0.3333333333333333703, 0.3333333333333333703, 0.3333333333333333703, 0.3333333333333333703, 0.3333333333333333703, 0.3333333333333333703),
 ( 0.3333333333333333703, 0.3333333333333333703, 0.3333333333333333703, 0.3333333333333333703, 0.3333333333333333703, 0.3333333333333333703, 0.3333333333333333703, 0.3333333333333333703, 0.3333333333333333703, 0.3333333333333333703, 0.3333333333333333703, 0.3333333333333333703, 0.3333333333333333703, 0.3333333333333333703, 0.3333333333333333703, 0.3333333333333333703, 0.3333333333333333703, 0.3333333333333333703, 0.3333333333333333703, 0.3333333333333333703, 0.3333333333333333703, 0.3333333333333333703, 0.3333333333333333703, 0.3333333333333333703, 0.3333333333333333703, 0.3333333333333333703, 0.3333333333333333703, 0.3333333333333333703, 0.3333333333333333703, 0.3333333333333333703),
 ( 1.000000000000000000, 1.000000000000000000, 1.000000000000000000, 1.000000000000000000, 1.000000000000000000, 1.000000000000000000, 1.000000000000000000, 1.000000000000000000, 1.000000000000000000, 1.000000000000000000, 1.000000000000000000, 1.000000000000000000, 1.000000000000000000, 1.000000000000000000, 1.000000000000000000, 1.000000000000000000, 1.000000000000000000, 1.000000000000000000, 1.000000000000000000, 1.000000000000000000, 1.000000000000000000, 1.000000000000000000, 1.000000000000000000, 1.000000000000000000, 1.000000000000000000, 1.000000000000000000, 1.000000000000000000, 1.000000000000000000, 1.000000000000000000, 1.000000000000000000),
 ( 0.3333333333333333703, 0.3333333333333333703, 0.3333333333333333703, 0.3333333333333333703, 0.3333333333333333703, 0.3333333333333333703, 0.3333333333333333703, 0.3333333333333333703, 0.3333333333333333703, 0.3333333333333333703, 0.3333333333333333703, 0.3333333333333333703, 0.3333333333333333703, 0.3333333333333333703, 0.3333333333333333703, 0.3333333333333333703, 0.3333333333333333703, 0.3333333333333333703, 0.3333333333333333703, 0.3333333333333333703, 0.3333333333333333703, 0.3333333333333333703, 0.3333333333333333703, 0.3333333333333333703, 0.3333333333333333703, 0.3333333333333333703, 0.3333333333333333703, 0.3333333333333333703, 0.3333333333333333703, 0.3333333333333333703),
 ( 0.3333333333333333703, 0.3333333333333333703, 0.3333333333333333703, 0.3333333333333333703, 0.3333333333333333703, 0.3333333333333333703, 0.3333333333333333703, 0.3333333333333333703, 0.3333333333333333703, 0.3333333333333333703, 0.3333333333333333703, 0.3333333333333333703, 0.3333333333333333703, 0.3333333333333333703, 0.3333333333333333703, 0.3333333333333333703, 0.3333333333333333703, 0.3333333333333333703, 0.3333333333333333703, 0.3333333333333333703, 0.3333333333333333703, 0.3333333333333333703, 0.3333333333333333703, 0.3333333333333333703, 0.3333333333333333703, 0.3333333333333333703, 0.3333333333333333703, 0.3333333333333333703, 0.3333333333333333703, 0.3333333333333333703),
 ( 1.000000000000000000, 1.000000000000000000, 1.000000000000000000, 1.000000000000000000, 1.000000000000000000, 1.000000000000000000, 1.000000000000000000, 1.000000000000000000, 1.000000000000000000, 1.000000000000000000, 1.000000000000000000, 1.000000000000000000, 1.000000000000000000, 1.000000000000000000, 1.000000000000000000, 1.000000000000000000, 1.000000000000000000, 1.000000000000000000, 1.000000000000000000, 1.000000000000000000, 1.000000000000000000, 1.000000000000000000, 1.000000000000000000, 1.000000000000000000, 1.000000000000000000, 1.000000000000000000, 1.000000000000000000, 1.000000000000000000, 1.000000000000000000, 1.000000000000000000) ) ) 
 REPRESENTATION_ITEM ( '' )  SURFACE ( )  );
#23374=CARTESIAN_POINT ( 'NONE',  ( 199.9999999999999432, -7.567711247534615993, 17.44155761536767812 ) ) ;
#23400=CARTESIAN_POINT ( 'NONE',  ( 200.0000000000000284, -3.097043465352568248, -18.74877632928372151 ) ) ;
#23404=CARTESIAN_POINT ( 'NONE',  ( 199.0053210531128229, 14.60061869579413063, -13.67646033072836786 ) ) ;
#23418=CARTESIAN_POINT ( 'NONE',  ( -135.8532207217289738, 21.81201906317729566, 34.75652343174635917 ) ) ;
#23430=CARTESIAN_POINT ( 'NONE',  ( 199.9999999999999716, 2.158921371974932057, 18.88613560767030464 ) ) ;
#23463=CARTESIAN_POINT ( 'NONE',  ( 199.0199467956651063, -18.45968165710057107, -7.701887558844384252 ) ) ;
#23473=CARTESIAN_POINT ( 'NONE',  ( 200.0000000000000000, -18.09920287623689106, -5.808051173427421610 ) ) ;
#23496=CARTESIAN_POINT ( 'NONE',  ( 199.9999999999998863, 8.252615397115851792, 17.12261885615216173 ) ) ;
#23521=CARTESIAN_POINT ( 'NONE',  ( 199.9999999999998295, -11.08011877867584261, -15.44095579151349185 ) ) ;
#23524=CARTESIAN_POINT ( 'NONE',  ( 199.0062091525825849, 18.60380424647159003, -7.335505861489442836 ) ) ;
#23553=CARTESIAN_POINT ( 'NONE',  ( 199.9999999999999147, 2.470466796131644660, 18.84784629003980783 ) ) ;
#23582=CARTESIAN_POINT ( 'NONE',  ( 199.0194986905590895, -18.08904332876870313, -8.539272476510683774 ) ) ;
#23590=CARTESIAN_POINT ( 'NONE',  ( 191.7822011676492195, 14.08373552998004463, -14.08373552997966449 ) ) ;
#23592=CARTESIAN_POINT ( 'NONE',  ( 200.0000000000000853, -18.97025941512468705, -1.247367644282773691 ) ) ;
#23618=CARTESIAN_POINT ( 'NONE',  ( 200.0000000000000284, 10.29196162618721644, 15.98165385515595815 ) ) ;
#23634=CARTESIAN_POINT ( 'NONE',  ( 136.1360204305621266, -24.77266263493151044, 24.77266263493093135 ) ) ;
#23645=CARTESIAN_POINT ( 'NONE',  ( 200.0000000000000853, -8.685123034760072969, -16.90575535186691880 ) ) ;
#23648=CARTESIAN_POINT ( 'NONE',  ( 199.0060120359516986, 18.22327268582330007, -8.235267977567980680 ) ) ;
#23667=CARTESIAN_POINT ( 'NONE',  ( 0.2972598230769938343, 10.13633138497486286, -10.13633138497461594 ) ) ;
#23671=ORIENTED_EDGE ( 'NONE', *, *, #14107, .F. ) ;
#23677=CARTESIAN_POINT ( 'NONE',  ( 199.0263554293247523, -15.04073044714995611, 13.19117051905602089 ) ) ;
#23707=CARTESIAN_POINT ( 'NONE',  ( 199.0159316777080676, -14.10546057009464072, -14.17879677899387758 ) ) ;
#23710=ORIENTED_EDGE ( 'NONE', *, *, #9807, .F. ) ;
#23717=CARTESIAN_POINT ( 'NONE',  ( 200.0000000000000284, -15.36457271445731543, -11.18861246136148502 ) ) ;
#23742=CARTESIAN_POINT ( 'NONE',  ( 199.9999999999999147, 2.470466796131644660, 18.84784629003980783 ) ) ;
#23758=CARTESIAN_POINT ( 'NONE',  ( 192.4448373802100889, -14.14213562375896061, 14.14213562375865330 ) ) ;
#23770=CARTESIAN_POINT ( 'NONE',  ( 200.0000000000000568, -16.61842928396364272, -9.229186156037545885 ) ) ;
#23774=CARTESIAN_POINT ( 'NONE',  ( 199.0054597862206549, 11.64633275074771035, -16.26583636099561403 ) ) ;
#23803=CARTESIAN_POINT ( 'NONE',  ( 199.9999999999997442, -9.911795474730137556, 16.22255894585034852 ) ) ;
#23833=CARTESIAN_POINT ( 'NONE',  ( 199.9999999999999432, 15.97944553385140587, -10.28395956944812362 ) ) ;
#23834=CARTESIAN_POINT ( 'NONE',  ( 199.0158433542230796, -13.98590299028042772, -14.29668655494494445 ) ) ;
#23876=CARTESIAN_POINT ( 'NONE',  ( 200.0000000000001137, 4.308913765035643273, 18.51575813813059668 ) ) ;
#23889=CARTESIAN_POINT ( 'NONE',  ( -91.56559293963834989, 40.53558337403654832, 16.03295912088756481 ) ) ;
#23905=CARTESIAN_POINT ( 'NONE',  ( 199.0072281836893637, 3.578240568248503894, -19.67355276342582115 ) ) ;
#23922=CARTESIAN_POINT ( 'NONE',  ( 146.6084372240433993, -24.48358557860353457, 24.48358557860296258 ) ) ;
#23933=CARTESIAN_POINT ( 'NONE',  ( 199.9999999999998863, 9.495902909754645904, 16.46521490772419583 ) ) ;
#23940=CARTESIAN_POINT ( 'NONE',  ( 57.59792236341147031, -1.722363176414363206, -54.84617931850881689 ) ) ;
#23943=CARTESIAN_POINT ( 'NONE',  ( -265.0000000000000000, -4.867971026610730343E-14, -6.532754371361504014E-30 ) ) ;
#23967=EDGE_LOOP ( 'NONE', ( #18305, #22087, #6919, #3888, #6733 ) ) ;
#23968=CARTESIAN_POINT ( 'NONE',  ( 199.9999999999999432, 18.99425342239354819, -0.6074896776222012962 ) ) ;
#23978=CARTESIAN_POINT ( 'NONE',  ( 146.6084372240433993, 3.800685668858732935, -3.800685668858610367 ) ) ;
#23980=CARTESIAN_POINT ( 'NONE',  ( 199.9999999999998579, -15.18157530797039101, 11.44282300742696457 ) ) ;
#23981=CARTESIAN_POINT ( 'NONE',  ( 199.0181823811410311, 10.83083347386195427, 16.81793973133765618 ) ) ;
#24008=CARTESIAN_POINT ( 'NONE',  ( 199.9999999999999716, 18.09021486607068496, 5.826594753398616433 ) ) ;
#24009=CARTESIAN_POINT ( 'NONE',  ( 199.9999999999999432, -18.36475088389829935, -4.912290392632249869 ) ) ;
#24012=ADVANCED_FACE ( 'NONE', ( #14868 ), #6886, .T. ) ;
#24021=CARTESIAN_POINT ( 'NONE',  ( 199.0154006451087128, 14.87427763521356461, 13.37117338753515305 ) ) ;
#24022=CARTESIAN_POINT ( 'NONE',  ( 151.7948205124836250, -23.49921654116371883, 23.49921654116317526 ) ) ;
#24039=CARTESIAN_POINT ( 'NONE',  ( 199.9999999999999147, -18.52330518485242195, -4.309840028370497400 ) ) ;
#24043=CARTESIAN_POINT ( 'NONE',  ( 199.0089689370622352, -1.315408825438062257, -19.96384840600867960 ) ) ;
#24072=CARTESIAN_POINT ( 'NONE',  ( 200.0000000000001421, 18.96284454896564142, 1.255519873078760229 ) ) ;
#24080=CARTESIAN_POINT ( 'NONE',  ( -208.1127848780264742, 10.60833733268383483, -67.17687982760675425 ) ) ;
#24108=CARTESIAN_POINT ( 'NONE',  ( 199.9999999999998863, 15.07162310294758711, 11.58087552627913119 ) ) ;
#24115=CARTESIAN_POINT ( 'NONE',  ( 199.0077026597514021, 2.114100997916472657, -19.88449140175694296 ) ) ;
#24125=CARTESIAN_POINT ( 'NONE',  ( 199.0222638060928375, 2.763249014911820733, 19.81200274180636711 ) ) ;
#24149=CARTESIAN_POINT ( 'NONE',  ( 199.9999999999998579, 17.67836847945686429, -6.970492097432807732 ) ) ;
#24150=CARTESIAN_POINT ( 'NONE',  ( 199.9999999999999432, -17.67796534906667816, -6.985163107940991267 ) ) ;
#24159=CARTESIAN_POINT ( 'NONE',  ( 199.0158545704749713, 14.28178091326991783, 14.00113215330521221 ) ) ;
#24161=CARTESIAN_POINT ( 'NONE',  ( 0.2972598230770011618, 10.13633138497555919, -66.70487387989845729 ) ) ;
#24174=CARTESIAN_POINT ( 'NONE',  ( 199.9999999999999716, -14.18957598410689869, 12.65210747703644500 ) ) ;
#24179=CARTESIAN_POINT ( 'NONE',  ( 199.0193324171001450, -17.94164708558885124, -8.847044913458905313 ) ) ;
#24211=CARTESIAN_POINT ( 'NONE',  ( 199.9999999999998010, 4.909892096549036467, 18.36538930945351566 ) ) ;
#24218=CARTESIAN_POINT ( 'NONE',  ( 170.2234770963711128, -17.36149277826940462, -39.20704971665412586 ) ) ;
#24219=CARTESIAN_POINT ( 'NONE',  ( 199.0225339954500328, 2.108197227390415929, 19.89250884296043864 ) ) ;
#24245=CARTESIAN_POINT ( 'NONE',  ( 199.9999999999999716, 18.74571404017359555, 3.115601181343412573 ) ) ;
#24251=CARTESIAN_POINT ( 'NONE',  ( 199.0112868605082497, -6.441215115722609852, -18.93473387006624620 ) ) ;
#24260=CARTESIAN_POINT ( 'NONE',  ( 199.0220573263155188, 3.250837537642027542, 19.73775173755759127 ) ) ;
#24289=AXIS2_PLACEMENT_3D ( 'NONE', #2436, #14659, #22799 ) ;
#24293=CARTESIAN_POINT ( 'NONE',  ( 199.9999999999999147, 16.22794370004292830, -9.883520089760141403 ) ) ;
#24295=CARTESIAN_POINT ( 'NONE',  ( 199.9999999999999432, -18.14801006015633789, 5.661042778411160548 ) ) ;
#24305=CARTESIAN_POINT ( 'NONE',  ( 199.0233413878889621, 0.01881827774306017026, 20.00361705477971341 ) ) ;
#24306=CARTESIAN_POINT ( 'NONE',  ( 170.2234770963711128, 39.20704971665372796, 17.36149277827039583 ) ) ;
#24308=CARTESIAN_POINT ( 'NONE',  ( -100.7734535825088500, 40.53558337403654832, 16.03295912088756481 ) ) ;
#24319=CARTESIAN_POINT ( 'NONE',  ( 200.0000000000000853, -18.00470042792477798, 6.107801588486966082 ) ) ;
#24322=CARTESIAN_POINT ( 'NONE',  ( 199.0104473268430922, -4.709499629590884417, -19.43548647772360383 ) ) ;
#24349=CARTESIAN_POINT ( 'NONE',  ( 199.9999999999998863, 14.88114354045644561, 11.82478185164094775 ) ) ;
#24355=CARTESIAN_POINT ( 'NONE',  ( -280.0000000000000568, -42.42640687119276066, -14.14213562373147148 ) ) ;
#24356=CARTESIAN_POINT ( 'NONE',  ( 199.0212010157159455, 5.167062836304152640, 19.32642926518865423 ) ) ;
#24380=CARTESIAN_POINT ( 'NONE',  ( 199.9999999999999716, 16.61865903285387347, -9.211533038762446779 ) ) ;
#24386=CARTESIAN_POINT ( 'NONE',  ( 199.0066734863077897, 5.484006884120094405, -19.23138624862535195 ) ) ;
#24395=CARTESIAN_POINT ( 'NONE',  ( 199.0158819412750688, 14.24569456864689343, 14.03872682698725249 ) ) ;
#24420=CARTESIAN_POINT ( 'NONE',  ( 199.9999999999999432, 17.03543292729471403, 8.423468753378063667 ) ) ;
#24421=CARTESIAN_POINT ( 'NONE',  ( 199.9999999999999147, -10.82661748099422638, -15.62198329103428840 ) ) ;
#24424=CARTESIAN_POINT ( 'NONE',  ( -280.0000000000000000, -5.143516556418885689E-14, 0.000000000000000000 ) ) ;
#24430=CARTESIAN_POINT ( 'NONE',  ( 199.0233313290092383, 0.04621523056493160447, 20.00358013886366138 ) ) ;
#24431=CARTESIAN_POINT ( 'NONE',  ( 57.59792236341147031, 54.84617931850878136, 1.722363176415705910 ) ) ;
#24433=CARTESIAN_POINT ( 'NONE',  ( 136.1360204305621551, 3.511608612530062512, 53.05693388239318864 ) ) ;
#24443=CARTESIAN_POINT ( 'NONE',  ( 200.0000000000000284, -19.00889450552964988, -0.1561390237190347086 ) ) ;
#24449=CARTESIAN_POINT ( 'NONE',  ( 199.0139917666041924, -11.25641580849352685, -16.53121693397544689 ) ) ;
#24481=CARTESIAN_POINT ( 'NONE',  ( 199.9999999999998579, 17.78360892267977178, 6.705045715290576247 ) ) ;
#24488=CARTESIAN_POINT ( 'NONE',  ( 200.0000000000000000, -42.42640687119272513, -14.14213562373140753 ) ) ;
#24489=CARTESIAN_POINT ( 'NONE',  ( 199.0216355752872914, 4.216131936211398035, 19.55614661669859444 ) ) ;
#24516=CARTESIAN_POINT ( 'NONE',  ( 199.9999999999999147, 7.543773257828894074, 17.44673522875667615 ) ) ;
#24523=CARTESIAN_POINT ( 'NONE',  ( 199.0122387307937686, -8.258478517853962586, -18.21619819090958714 ) ) ;
#24532=CARTESIAN_POINT ( 'NONE',  ( 199.0244464070843833, -3.263486543644114946, 19.73887645897787735 ) ) ;
#24557=CARTESIAN_POINT ( 'NONE',  ( 199.9999999999998863, 15.61930985130600291, 10.83040361559445230 ) ) ;
#24558=CARTESIAN_POINT ( 'NONE',  ( 200.0000000000000000, -10.30695654162946795, -15.96943722719255199 ) ) ;
#24567=CARTESIAN_POINT ( 'NONE',  ( 199.0233077721956647, 0.1102320784427082423, 20.00336233838309496 ) ) ;
#24568=CARTESIAN_POINT ( 'NONE',  ( 192.4448373802101173, 42.42640687116487896, 14.14213562375934075 ) ) ;
#24570=CARTESIAN_POINT ( 'NONE',  ( -162.0762913951021176, 29.48230308784730980, 27.08623940707652622 ) ) ;
#24582=CARTESIAN_POINT ( 'NONE',  ( 199.0100048860339541, -3.743224330709818748, -19.64425440907078269 ) ) ;
#24613=CARTESIAN_POINT ( 'NONE',  ( 200.0000000000001705, 5.211075256460824257, -18.27473396828003871 ) ) ;
#24619=CARTESIAN_POINT ( 'NONE',  ( 91.82158438592158234, -12.16597498397778843, 12.16597498397750954 ) ) ;
#24620=CARTESIAN_POINT ( 'NONE',  ( 199.0248683625651154, -4.715036670046848677, 19.44145415004932076 ) ) ;
#24652=CARTESIAN_POINT ( 'NONE',  ( 199.0103724725597658, -4.548822225537863417, -19.47368150598642345 ) ) ;
#24663=CARTESIAN_POINT ( 'NONE',  ( 199.0106735244355320, 19.32142130491951804, 5.196343561012195522 ) ) ;
#24677=CARTESIAN_POINT ( 'NONE',  ( 199.0129030236711003, -9.437255757388491872, -17.63982070750089548 ) ) ;
#24688=CARTESIAN_POINT ( 'NONE',  ( 200.0000000000002558, -1.250172057809772586, -18.97074946354465652 ) ) ;
#24690=CARTESIAN_POINT ( 'NONE',  ( 199.9999999999999147, 10.29454322937508159, -15.97255386245730691 ) ) ;
#24701=CARTESIAN_POINT ( 'NONE',  ( 199.0083531997975967, 19.99451597160352989, -0.2840371431019264592 ) ) ;
#24703=CARTESIAN_POINT ( 'NONE',  ( -135.8532207217289738, 21.81201906317798134, -21.81201906317747685 ) ) ;
#24705=CARTESIAN_POINT ( 'NONE',  ( -259.2033419157646676, 49.83842185052017015, 6.730120644404137487 ) ) ;
#24719=CARTESIAN_POINT ( 'NONE',  ( 199.0253131443098766, -18.94683372192476156, 6.427280041807147626 ) ) ;
#24747=CARTESIAN_POINT ( 'NONE',  ( 200.0000000000005116, 16.46820326627658204, -9.481692438271846157 ) ) ;
#24753=CARTESIAN_POINT ( 'NONE',  ( 192.4448373802100889, -14.14213562375896061, 14.14213562375865330 ) ) ;
#24754=CARTESIAN_POINT ( 'NONE',  ( 199.0261637166634330, -10.98746419350304748, 16.71832627740758070 ) ) ;
#24766=CARTESIAN_POINT ( 'NONE',  ( 199.0260481038674811, -10.14773143618404383, 17.24088832081764622 ) ) ;
#24787=CARTESIAN_POINT ( 'NONE',  ( 199.0248198352711313, -19.48551319141294869, 4.538181572781159190 ) ) ;
#24798=CARTESIAN_POINT ( 'NONE',  ( 199.0062801269303350, 18.72091001596172433, -7.031396878026334285 ) ) ;
#24811=CARTESIAN_POINT ( 'NONE',  ( 199.0079621347063892, 1.362236960746584069, -19.95249283290727860 ) ) ;
#24821=LINE ( 'NONE', #8711, #18575 ) ;
#24822=CARTESIAN_POINT ( 'NONE',  ( 199.9999999999998579, -2.482523633563583410, -18.84177167654976515 ) ) ;
#24824=CARTESIAN_POINT ( 'NONE',  ( 199.9999999999999147, 5.804186778207960806, -18.09503644758711260 ) ) ;
#24833=CARTESIAN_POINT ( 'NONE',  ( 199.0060273340149024, 18.25277364203476438, -8.166168630484282431 ) ) ;
#24834=CARTESIAN_POINT ( 'NONE',  ( -100.7734535825088500, -44.31723036834885932, -12.25131212657538171 ) ) ;
#24836=CARTESIAN_POINT ( 'NONE',  ( 192.4448373802101173, 14.14213562370261279, 42.42640687122091236 ) ) ;
#24849=CARTESIAN_POINT ( 'NONE',  ( 199.9999999999997442, -9.911795474730137556, 16.22255894585034852 ) ) ;
#24874=ORIENTED_EDGE ( 'NONE', *, *, #26231, .F. ) ;
#24878=CARTESIAN_POINT ( 'NONE',  ( 200.0000000000001137, 18.27430636540404407, -5.205727087885991367 ) ) ;
#24881=CARTESIAN_POINT ( 'NONE',  ( -162.0762913951020892, 1.198031840385732849, -1.198031840385733515 ) ) ;
#24882=CARTESIAN_POINT ( 'NONE',  ( 199.0120816426991155, 18.34336195414084969, 7.966874786652939910 ) ) ;
#24897=CARTESIAN_POINT ( 'NONE',  ( 199.0263607205240532, -13.20175300279655062, 15.04466839055514527 ) ) ;
#24914=CARTESIAN_POINT ( 'NONE',  ( 199.9999999999999716, 3.394816402666279931, 18.70522384341381894 ) ) ;
#24920=CARTESIAN_POINT ( 'NONE',  ( 199.0178460907175690, -16.45326163792621443, -11.37340206338170923 ) ) ;
#24934=CARTESIAN_POINT ( 'NONE',  ( 199.0125740919301336, 17.92725630381683644, 8.864156431172764528 ) ) ;
#24952=CARTESIAN_POINT ( 'NONE',  ( 199.0056803851548750, 10.03079491058490724, -17.30956630377439254 ) ) ;
#24963=CARTESIAN_POINT ( 'NONE',  ( 200.0000000000000284, 15.35911892145054303, -11.18589804280325772 ) ) ;
#24973=CARTESIAN_POINT ( 'NONE',  ( 199.0084097827293590, 19.99587590986774188, -0.1328658178166673143 ) ) ;
#24974=CARTESIAN_POINT ( 'NONE',  ( -135.8532207217289738, -6.472252184284280396, 6.472252184284099208 ) ) ;
#24988=CARTESIAN_POINT ( 'NONE',  ( 199.0263356842403653, -15.36141226383640301, 12.81629321302553848 ) ) ;
#25014=CARTESIAN_POINT ( 'NONE',  ( 200.0000000000000000, 17.99825158093497635, -6.097534595090909448 ) ) ;
#25017=CARTESIAN_POINT ( 'NONE',  ( -198.0356074513804572, -17.40982414986427429, -39.15871834505933435 ) ) ;
#25018=CARTESIAN_POINT ( 'NONE',  ( 199.0135736376541615, 16.97384353125803003, 10.58053792802146020 ) ) ;
#25048=CARTESIAN_POINT ( 'NONE',  ( 200.0000000000000284, 4.759886302454138018, 18.40685213041688328 ) ) ;
#25053=CARTESIAN_POINT ( 'NONE',  ( 199.0179304339989415, -16.54579169021749863, -11.23843401478282544 ) ) ;
#25064=CARTESIAN_POINT ( 'NONE',  ( 199.0087145623001277, 19.98798542585446469, 0.6659850717246563745 ) ) ;
#25079=CARTESIAN_POINT ( 'NONE',  ( 199.0061245020890510, 7.715982321041501280, -18.44633997128330805 ) ) ;
#25086=ADVANCED_FACE ( 'NONE', ( #22638 ), #19316, .F. ) ;
#25094=CARTESIAN_POINT ( 'NONE',  ( 199.9999999999999147, -3.403913688674531812, -18.69557029314349705 ) ) ;
#25096=CARTESIAN_POINT ( 'NONE',  ( 199.9999999999999147, 7.548244939093340378, -17.43950459141031573 ) ) ;
#25104=CARTESIAN_POINT ( 'NONE',  ( 199.0075046806690295, 19.82372177647270917, -2.703293726033221045 ) ) ;
#25105=CARTESIAN_POINT ( 'NONE',  ( 0.2972598230769938343, 10.13633138497486286, -10.13633138497461594 ) ) ;
#25119=CARTESIAN_POINT ( 'NONE',  ( 199.0203632001705216, -18.77805633539013996, -6.891912269405206182 ) ) ;
#25144=ORIENTED_EDGE ( 'NONE', *, *, #25405, .T. ) ;
#25147=CARTESIAN_POINT ( 'NONE',  ( 199.9999999999998863, 18.88157209772827017, -2.150785294275829429 ) ) ;
#25151=CARTESIAN_POINT ( 'NONE',  ( 199.0188463327468185, 9.707946089746242180, 17.48826952134088941 ) ) ;
#25166=CARTESIAN_POINT ( 'NONE',  ( 192.4448373802100889, -14.14213562375896061, 14.14213562375865330 ) ) ;
#25178=CARTESIAN_POINT ( 'NONE',  ( 199.9999999999998863, -1.253919976928773661, 19.00818551405020784 ) ) ;
#25182=PRODUCT_DEFINITION ( 'UNKNOWN', '', #12999, #13227 ) ;
#25184=CARTESIAN_POINT ( 'NONE',  ( 199.0201284062958962, -18.60237515726647572, -7.352601386804158423 ) ) ;
#25197=CARTESIAN_POINT ( 'NONE',  ( 199.0117592729713465, 18.59672480091233737, 7.361113620700817428 ) ) ;
#25206=ORIENTED_EDGE ( 'NONE', *, *, #19215, .F. ) ;
#25212=CARTESIAN_POINT ( 'NONE',  ( 199.0105764394585890, -4.988040173753162776, -19.37759405569597959 ) ) ;
#25220=CARTESIAN_POINT ( 'NONE',  ( 199.9999999999999147, 1.697088945475840660, -18.92594139730135439 ) ) ;
#25221=CARTESIAN_POINT ( 'NONE',  ( 200.0000000000000000, 9.228668854417362510, -16.61132610550090760 ) ) ;
#25231=CARTESIAN_POINT ( 'NONE',  ( 57.59792236341147031, -1.722363176414363206, -54.84617931850881689 ) ) ;
#25245=CARTESIAN_POINT ( 'NONE',  ( 199.0234688043258018, -20.00162938710794691, 0.3307560783973806373 ) ) ;
#25274=CARTESIAN_POINT ( 'NONE',  ( 200.0000000000001705, -16.91021041590709473, -8.683373960011902426 ) ) ;
#25278=CARTESIAN_POINT ( 'NONE',  ( 199.0116003924211725, 18.71458825927322422, 7.055789865482638312 ) ) ;
#25291=CARTESIAN_POINT ( 'NONE',  ( 199.0256575778758474, -7.963596585350240176, 18.35421432800287533 ) ) ;
#25293=CARTESIAN_POINT ( 'NONE',  ( -208.1127848780264742, 67.17687982763172272, -10.60833733270698254 ) ) ;
#25308=CARTESIAN_POINT ( 'NONE',  ( 199.9999999999999716, -3.868950841772955673, 18.61236034055575317 ) ) ;
#25337=ORIENTED_EDGE ( 'NONE', *, *, #17104, .T. ) ;
#25340=CARTESIAN_POINT ( 'NONE',  ( 199.0232538779058302, -20.00218003532801703, -0.2559617245760326676 ) ) ;
#25350=CARTESIAN_POINT ( 'NONE',  ( 200.0000000000000000, -14.79283710360616944, -11.93388616463377438 ) ) ;
#25363=CARTESIAN_POINT ( 'NONE',  ( 19.06497207195981858, 10.03556273973516078, -66.60410523465806421 ) ) ;
#25379=CARTESIAN_POINT ( 'NONE',  ( 200.0000000000000000, -3.101357108925543837, 18.75734389255849521 ) ) ;
#25403=CARTESIAN_POINT ( 'NONE',  ( 200.0000000000001137, -16.46591192518303970, -9.498466322123544359 ) ) ;
#25405=EDGE_CURVE ( 'NONE', #13305, #20820, #18832, .T. ) ;
#25406=CARTESIAN_POINT ( 'NONE',  ( 199.0076515966382260, 19.86999350167783263, -2.263549309587763680 ) ) ;
#25423=CARTESIAN_POINT ( 'NONE',  ( -208.1127848780264742, 38.89260858015707356, 17.67593391476696141 ) ) ;
#25438=CARTESIAN_POINT ( 'NONE',  ( 199.9999999999999147, -9.100092698529554269, 16.69133291234032868 ) ) ;
#25478=CARTESIAN_POINT ( 'NONE',  ( -238.4067589809705794, 28.96627169325354956, -28.96627169325289231 ) ) ;
#25480=CARTESIAN_POINT ( 'NONE',  ( 199.9999999999999147, -18.52330518485242195, -4.309840028370497400 ) ) ;
#25505=CARTESIAN_POINT ( 'NONE',  ( 199.9999999999999147, 6.094537134382843391, 18.00666549647224812 ) ) ;
#25532=CARTESIAN_POINT ( 'NONE',  ( 200.0000000000000284, -15.36457271445731543, -11.18861246136148502 ) ) ;
#25535=CARTESIAN_POINT ( 'NONE',  ( 199.0076473327615645, 2.278485796641462446, -19.86629856447459375 ) ) ;
#25565=CARTESIAN_POINT ( 'NONE',  ( 199.0262887415137527, -15.87643591937917442, 12.17243215972436055 ) ) ;
#25596=CARTESIAN_POINT ( 'NONE',  ( 199.0189539020448990, -17.60163767500414522, -9.515575210798317585 ) ) ;
#25607=CARTESIAN_POINT ( 'NONE',  ( 163.1118516004056573, 9.006482792069759213, -9.006482792069505194 ) ) ;
#25609=CARTESIAN_POINT ( 'NONE',  ( 200.0000000000000568, -16.61842928396364272, -9.229186156037545885 ) ) ;
#25633=CARTESIAN_POINT ( 'NONE',  ( 200.0000000000005684, -1.253076495463282924, 18.97792690268338234 ) ) ;
#25657=CARTESIAN_POINT ( 'NONE',  ( 199.9999999999999432, -9.907006709245502307, -16.21817530592209522 ) ) ;
#25660=CARTESIAN_POINT ( 'NONE',  ( 199.0066734863077897, 5.484006884120094405, -19.23138624862535195 ) ) ;
#25678=CARTESIAN_POINT ( 'NONE',  ( -30.26275506840324070, 1.198031551616030033, -1.198031551616006496 ) ) ;
#25688=CARTESIAN_POINT ( 'NONE',  ( 199.9999999999998010, -6.124229907523811356, 17.99904841416608292 ) ) ;
#25713=CARTESIAN_POINT ( 'NONE',  ( 199.0263771353515949, -14.14574067859894413, 14.14574067859863682 ) ) ;
#25716=CARTESIAN_POINT ( 'NONE',  ( 199.0255773684291967, -18.50957944509308462, 7.588431196845307980 ) ) ;
#25727=CARTESIAN_POINT ( 'NONE',  ( 200.0000000000000284, -8.407999580957739028, -17.04516676560209376 ) ) ;
#25761=CARTESIAN_POINT ( 'NONE',  ( 199.9999999999998863, -9.236595569432955344, 16.61620204157069125 ) ) ;
#25774=CARTESIAN_POINT ( 'NONE',  ( 151.7948205124836250, -23.49921654116371883, 23.49921654116317526 ) ) ;
#25784=CARTESIAN_POINT ( 'NONE',  ( 199.9999999999998295, -7.847915761074617080, -17.31000481134407565 ) ) ;
#25787=CARTESIAN_POINT ( 'NONE',  ( 199.0073354103614918, 19.73522450985164411, -3.233483297802316692 ) ) ;
#25819=CARTESIAN_POINT ( 'NONE',  ( 199.9999999999999147, -11.82758851212937579, 14.88619241608240529 ) ) ;
#25852=CARTESIAN_POINT ( 'NONE',  ( 199.9999999999999716, 14.31544119637113432, -12.55530011466301055 ) ) ;
#25853=CARTESIAN_POINT ( 'NONE',  ( 199.0157566623909702, -13.86784264559070756, -14.41179826723872459 ) ) ;
#25863=CARTESIAN_POINT ( 'NONE',  ( 199.9999999999998863, -11.20618975336454071, -15.34975362513495689 ) ) ;
#25892=CARTESIAN_POINT ( 'NONE',  ( 199.9999999999999432, 3.548988777896260771, 18.67457114543681485 ) ) ;
#25905=CARTESIAN_POINT ( 'NONE',  ( -213.1075012329537230, 66.26714140138673770, -9.698598906462034819 ) ) ;
#25918=CARTESIAN_POINT ( 'NONE',  ( 200.0000000000000568, -14.79650836250383250, 11.93661649116771173 ) ) ;
#25922=AXIS2_PLACEMENT_3D ( 'NONE', #19385, #19260, #16999 ) ;
#25924=CARTESIAN_POINT ( 'NONE',  ( 199.0060751070798233, 18.35498561216385482, -7.937441424495496278 ) ) ;
#25943=CARTESIAN_POINT ( 'NONE',  ( 184.5754832356733459, -14.84877008830847345, 14.84877008830815015 ) ) ;
#25954=CARTESIAN_POINT ( 'NONE',  ( 199.9999999999998295, 13.96930097052764097, 12.88701297307445159 ) ) ;
#25960=CARTESIAN_POINT ( 'NONE',  ( -213.1075012329537230, 9.698598906438871126, -66.26714140136179765 ) ) ;
#26000=CARTESIAN_POINT ( 'NONE',  ( 130.8568914410475372, 4.207082182992923691, -4.207082182992794017 ) ) ;
#26004=CARTESIAN_POINT ( 'NONE',  ( 199.0249556294982938, -5.033924301686514724, 19.36137939705603017 ) ) ;
#26030=CARTESIAN_POINT ( 'NONE',  ( 199.9999999999998579, 18.35745069958362308, -4.904641354906189576 ) ) ;
#26031=CARTESIAN_POINT ( 'NONE',  ( 200.0000000000000000, -17.61921750228558281, -7.131901422850258854 ) ) ;
#26042=CARTESIAN_POINT ( 'NONE',  ( 184.8905102610680444, 13.49065550809757497, 43.07788698682593065 ) ) ;
#26045=CARTESIAN_POINT ( 'NONE',  ( -238.4067589809705794, 28.96627169325285678, 27.60227080167094726 ) ) ;
#26057=CARTESIAN_POINT ( 'NONE',  ( 199.0074854128475579, 2.768696461275208520, -19.80384161416936806 ) ) ;
#26080=MANIFOLD_SOLID_BREP ( 'Chamfer3', #4528 ) ;
#26088=CARTESIAN_POINT ( 'NONE',  ( 200.0000000000001421, 9.088304224312857116, 16.69380151103622012 ) ) ;
#26095=CARTESIAN_POINT ( 'NONE',  ( -213.1075012329537230, 37.98287015391280619, -37.98287015391192512 ) ) ;
#26119=CARTESIAN_POINT ( 'NONE',  ( 199.9999999999999432, 18.94174490274730616, -1.534455786497347596 ) ) ;
#26125=CARTESIAN_POINT ( 'NONE',  ( 199.0125641721520822, -8.847877585088737007, -17.93749959268865979 ) ) ;
#26134=CARTESIAN_POINT ( 'NONE',  ( 199.0132385929227610, 17.30986399168244461, 10.02103235953326710 ) ) ;
#26156=CIRCLE ( 'NONE', #14668, 10.00000000000000000 ) ;
#26161=EDGE_CURVE ( 'NONE', #21338, #13305, #1349, .T. ) ;
#26164=CARTESIAN_POINT ( 'NONE',  ( 199.9999999999999432, 14.48708306876533136, 12.30466461812483914 ) ) ;
#26166=CARTESIAN_POINT ( 'NONE',  ( 199.9999999999999716, -18.97839083694794837, 1.248491631922335143 ) ) ;
#26176=CARTESIAN_POINT ( 'NONE',  ( 199.0229061757917464, 1.171229046118675177, 19.97135794441219048 ) ) ;
#26178=CARTESIAN_POINT ( 'NONE',  ( -86.96347745069644475, -15.38646221621738164, -41.18208027870615240 ) ) ;
#26182=CARTESIAN_POINT ( 'NONE',  ( -56.48582580120559271, -6.472252184284276844, 6.472252184284108978 ) ) ;
#26195=CARTESIAN_POINT ( 'NONE',  ( 199.9999999999998295, -17.79330310134281135, 6.698924172861754123 ) ) ;
#26199=CARTESIAN_POINT ( 'NONE',  ( 199.0142478014330720, -11.65985798941387941, -16.24932773989132073 ) ) ;
#26228=CARTESIAN_POINT ( 'NONE',  ( 199.9999999999998579, 13.31531350134012648, 13.56203446005050317 ) ) ;
#26231=EDGE_CURVE ( 'NONE', #122, #5454, #8298, .T. ) ;
#26235=CARTESIAN_POINT ( 'NONE',  ( -105.3755690713226727, 12.89780903124418998, -12.89780903124389155 ) ) ;
#26236=CARTESIAN_POINT ( 'NONE',  ( 199.0261090282319856, -10.57113834583376644, 16.98461103275367634 ) ) ;
#26261=CARTESIAN_POINT ( 'NONE',  ( 199.9999999999999432, 17.67867420253430311, -6.969775622007540861 ) ) ;
#26268=CARTESIAN_POINT ( 'NONE',  ( 199.0083412756643497, 0.3136196654984919618, -19.99640146592421175 ) ) ;
#26277=CARTESIAN_POINT ( 'NONE',  ( 199.0247325273615502, -4.232801689760709252, 19.55205092890061280 ) ) ;
#26299=CARTESIAN_POINT ( 'NONE',  ( 199.0053211804427633, 14.13331159297750617, -14.14343255912447361 ) ) ;
#26300=CARTESIAN_POINT ( 'NONE',  ( 199.9999999999998863, 18.97179924413623908, -1.226483293096950700 ) ) ;
#26301=CARTESIAN_POINT ( 'NONE',  ( 199.9999999999999147, -17.95406390809352004, -6.253787172257868399 ) ) ;
#26312=CARTESIAN_POINT ( 'NONE',  ( -213.1075012329537230, 37.98287015391280619, -37.98287015391192512 ) ) ;
#26324=CARTESIAN_POINT ( 'NONE',  ( 200.0000000000001990, -15.46007656673369368, 11.06691610098113543 ) ) ;
#26329=CARTESIAN_POINT ( 'NONE',  ( 199.0122387307937686, -8.258478517853962586, -18.21619819090958714 ) ) ;
#26403=COLOUR_RGB('Off White',0.89,0.88,0.83);
#26404=FILL_AREA_STYLE_COLOUR('',#26403);
#26405=FILL_AREA_STYLE('',(#26404));
#26406=SURFACE_STYLE_FILL_AREA(#26405);
#26407=SURFACE_SIDE_STYLE('',(#26406));
#26408=SURFACE_STYLE_USAGE(.BOTH.,#26407);
#26409=PRESENTATION_STYLE_ASSIGNMENT((#26408));
ENDSEC;
END-ISO-10303-21;
